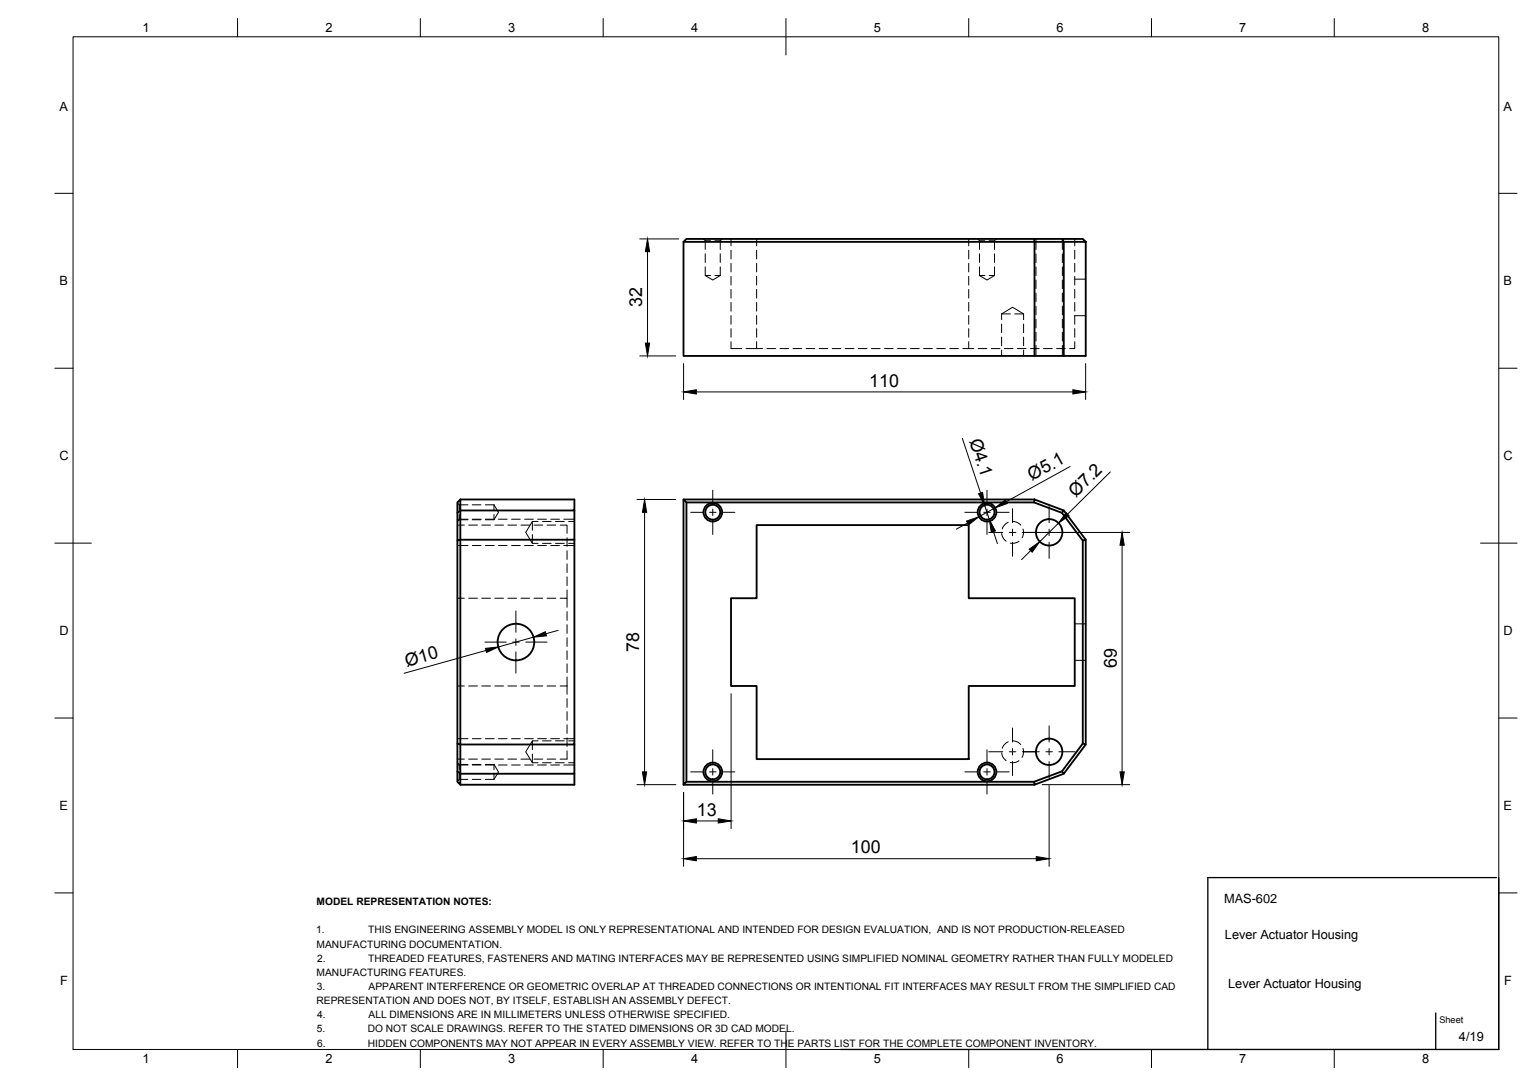
ISO-10303-21;
HEADER;
/* Generated by software containing ST-Developer
 * from STEP Tools, Inc. (www.steptools.com) 
 */

FILE_DESCRIPTION(
/* description */ (''),
/* implementation_level */ '2;1');

FILE_NAME(
/* name */ 'Lever Actuator Housing.step',
/* time_stamp */ '2026-10-15T14:42:47-07:00',
/* author */ (''),
/* organization */ (''),
/* preprocessor_version */ 'ST-DEVELOPER v20.2',
/* originating_system */ 'Autodesk Translation Framework v15.15.0.0',
/* authorisation */ '');

FILE_SCHEMA (('AUTOMOTIVE_DESIGN { 1 0 10303 214 3 1 1 }'));
ENDSEC;

DATA;
#10=MECHANICAL_DESIGN_GEOMETRIC_PRESENTATION_REPRESENTATION('',(#235),#85789);
#153=CONICAL_SURFACE('',#10323,0.1025,1.02974425867665);
#154=CONICAL_SURFACE('',#10327,0.255,0.785398163397446);
#155=CONICAL_SURFACE('',#10328,0.1025,1.02974425867665);
#156=CONICAL_SURFACE('',#10332,0.255,0.785398163397448);
#157=CONICAL_SURFACE('',#10333,0.1025,1.02974425867665);
#158=CONICAL_SURFACE('',#10337,0.255,0.785398163397446);
#159=CONICAL_SURFACE('',#10338,0.1025,1.02974425867665);
#160=CONICAL_SURFACE('',#10342,0.255,0.785398163397448);
#161=CONICAL_SURFACE('',#10343,0.15,1.02974425867665);
#162=CONICAL_SURFACE('',#10347,0.15,1.02974425867665);
#199=SHAPE_REPRESENTATION_RELATIONSHIP('SRR','None',#85864,#217);
#217=ADVANCED_BREP_SHAPE_REPRESENTATION('',(#253),#85772);
#235=STYLED_ITEM('',(#85963),#253);
#253=MANIFOLD_SOLID_BREP('Body1',#9882);
#398=FACE_BOUND('',#3084,.T.);
#399=FACE_BOUND('',#3085,.T.);
#400=FACE_BOUND('',#3086,.T.);
#401=FACE_BOUND('',#3087,.T.);
#402=FACE_BOUND('',#3088,.T.);
#403=FACE_BOUND('',#3089,.T.);
#404=FACE_BOUND('',#3090,.T.);
#405=FACE_BOUND('',#3114,.T.);
#406=FACE_BOUND('',#3126,.T.);
#407=FACE_BOUND('',#3130,.T.);
#408=FACE_BOUND('',#3131,.T.);
#409=FACE_BOUND('',#3132,.T.);
#410=FACE_BOUND('',#3133,.T.);
#1013=PLANE('',#10304);
#1014=PLANE('',#10305);
#1015=PLANE('',#10306);
#1016=PLANE('',#10307);
#1017=PLANE('',#10308);
#1018=PLANE('',#10309);
#1019=PLANE('',#10310);
#1020=PLANE('',#10311);
#1021=PLANE('',#10312);
#1022=PLANE('',#10313);
#1023=PLANE('',#10314);
#1024=PLANE('',#10315);
#1025=PLANE('',#10316);
#1026=PLANE('',#10358);
#1027=PLANE('',#10359);
#1028=PLANE('',#10360);
#1029=PLANE('',#10361);
#1030=PLANE('',#10362);
#1031=PLANE('',#10363);
#1032=PLANE('',#10364);
#1033=PLANE('',#10365);
#1034=PLANE('',#10366);
#1035=PLANE('',#10367);
#1036=PLANE('',#10368);
#1037=PLANE('',#10369);
#1038=PLANE('',#10370);
#1039=PLANE('',#10371);
#1040=PLANE('',#10372);
#1041=PLANE('',#10373);
#1042=PLANE('',#10374);
#1043=PLANE('',#10375);
#1262=LINE('',#23334,#1798);
#1263=LINE('',#23336,#1799);
#1264=LINE('',#23338,#1800);
#1265=LINE('',#23339,#1801);
#1266=LINE('',#23342,#1802);
#1267=LINE('',#23344,#1803);
#1268=LINE('',#23345,#1804);
#1269=LINE('',#23348,#1805);
#1270=LINE('',#23350,#1806);
#1271=LINE('',#23351,#1807);
#1272=LINE('',#23354,#1808);
#1273=LINE('',#23356,#1809);
#1274=LINE('',#23357,#1810);
#1275=LINE('',#23360,#1811);
#1276=LINE('',#23362,#1812);
#1277=LINE('',#23363,#1813);
#1278=LINE('',#23366,#1814);
#1279=LINE('',#23368,#1815);
#1280=LINE('',#23369,#1816);
#1281=LINE('',#23372,#1817);
#1282=LINE('',#23374,#1818);
#1283=LINE('',#23375,#1819);
#1284=LINE('',#23377,#1820);
#1285=LINE('',#23378,#1821);
#1286=LINE('',#23381,#1822);
#1287=LINE('',#23383,#1823);
#1288=LINE('',#23384,#1824);
#1289=LINE('',#23387,#1825);
#1290=LINE('',#23388,#1826);
#1291=LINE('',#23391,#1827);
#1292=LINE('',#23392,#1828);
#1293=LINE('',#23395,#1829);
#1294=LINE('',#23396,#1830);
#1295=LINE('',#23400,#1831);
#1296=LINE('',#23402,#1832);
#1297=LINE('',#23404,#1833);
#1298=LINE('',#23406,#1834);
#1299=LINE('',#23408,#1835);
#1300=LINE('',#23410,#1836);
#1301=LINE('',#23412,#1837);
#1302=LINE('',#23414,#1838);
#1303=LINE('',#23416,#1839);
#1304=LINE('',#23418,#1840);
#1305=LINE('',#23420,#1841);
#1306=LINE('',#23421,#1842);
#1307=LINE('',#23437,#1843);
#1308=LINE('',#23441,#1844);
#1309=LINE('',#23444,#1845);
#1310=LINE('',#23448,#1846);
#1311=LINE('',#23452,#1847);
#1312=LINE('',#23455,#1848);
#1313=LINE('',#23459,#1849);
#1314=LINE('',#23463,#1850);
#1315=LINE('',#23466,#1851);
#1316=LINE('',#23470,#1852);
#1317=LINE('',#23474,#1853);
#1318=LINE('',#23477,#1854);
#1319=LINE('',#23481,#1855);
#1320=LINE('',#23485,#1856);
#1321=LINE('',#23490,#1857);
#1322=LINE('',#23494,#1858);
#1323=LINE('',#23499,#1859);
#1324=LINE('',#23503,#1860);
#1325=LINE('',#23508,#1861);
#1326=LINE('',#23512,#1862);
#1327=LINE('',#23514,#1863);
#1328=LINE('',#23515,#1864);
#1329=LINE('',#23518,#1865);
#1330=LINE('',#23519,#1866);
#1331=LINE('',#23522,#1867);
#1332=LINE('',#23523,#1868);
#1333=LINE('',#23526,#1869);
#1334=LINE('',#23527,#1870);
#1335=LINE('',#23530,#1871);
#1336=LINE('',#23531,#1872);
#1337=LINE('',#23534,#1873);
#1338=LINE('',#23535,#1874);
#1339=LINE('',#23538,#1875);
#1340=LINE('',#23539,#1876);
#1341=LINE('',#23542,#1877);
#1342=LINE('',#23543,#1878);
#1343=LINE('',#23546,#1879);
#1344=LINE('',#23547,#1880);
#1345=LINE('',#23550,#1881);
#1346=LINE('',#23551,#1882);
#1347=LINE('',#23554,#1883);
#1348=LINE('',#23555,#1884);
#1349=LINE('',#23557,#1885);
#1350=LINE('',#23561,#1886);
#1351=LINE('',#23562,#1887);
#1352=LINE('',#23565,#1888);
#1353=LINE('',#23566,#1889);
#1354=LINE('',#23569,#1890);
#1355=LINE('',#23570,#1891);
#1356=LINE('',#23572,#1892);
#1798=VECTOR('',#11436,1.);
#1799=VECTOR('',#11437,1.);
#1800=VECTOR('',#11438,1.);
#1801=VECTOR('',#11439,0.999999999999999);
#1802=VECTOR('',#11442,1.);
#1803=VECTOR('',#11443,1.);
#1804=VECTOR('',#11444,1.);
#1805=VECTOR('',#11447,1.);
#1806=VECTOR('',#11448,1.);
#1807=VECTOR('',#11449,1.);
#1808=VECTOR('',#11452,1.);
#1809=VECTOR('',#11453,1.);
#1810=VECTOR('',#11454,1.);
#1811=VECTOR('',#11457,1.);
#1812=VECTOR('',#11458,1.);
#1813=VECTOR('',#11459,1.);
#1814=VECTOR('',#11462,1.);
#1815=VECTOR('',#11463,1.);
#1816=VECTOR('',#11464,1.);
#1817=VECTOR('',#11467,1.);
#1818=VECTOR('',#11468,1.);
#1819=VECTOR('',#11469,1.);
#1820=VECTOR('',#11472,1.);
#1821=VECTOR('',#11473,1.);
#1822=VECTOR('',#11476,1.);
#1823=VECTOR('',#11477,1.);
#1824=VECTOR('',#11478,1.);
#1825=VECTOR('',#11481,1.);
#1826=VECTOR('',#11482,1.);
#1827=VECTOR('',#11485,1.);
#1828=VECTOR('',#11486,1.);
#1829=VECTOR('',#11489,1.);
#1830=VECTOR('',#11490,1.);
#1831=VECTOR('',#11493,1.);
#1832=VECTOR('',#11494,1.);
#1833=VECTOR('',#11495,1.);
#1834=VECTOR('',#11496,1.);
#1835=VECTOR('',#11497,1.);
#1836=VECTOR('',#11498,1.);
#1837=VECTOR('',#11499,1.);
#1838=VECTOR('',#11500,1.);
#1839=VECTOR('',#11501,1.);
#1840=VECTOR('',#11502,1.);
#1841=VECTOR('',#11503,1.);
#1842=VECTOR('',#11504,1.);
#1843=VECTOR('',#11519,0.1025);
#1844=VECTOR('',#11524,0.205);
#1845=VECTOR('',#11529,0.255);
#1846=VECTOR('',#11532,0.1025);
#1847=VECTOR('',#11537,0.205);
#1848=VECTOR('',#11542,0.255);
#1849=VECTOR('',#11545,0.1025);
#1850=VECTOR('',#11550,0.205);
#1851=VECTOR('',#11555,0.255);
#1852=VECTOR('',#11558,0.1025);
#1853=VECTOR('',#11563,0.205);
#1854=VECTOR('',#11568,0.255);
#1855=VECTOR('',#11571,0.15);
#1856=VECTOR('',#11576,0.3);
#1857=VECTOR('',#11581,0.15);
#1858=VECTOR('',#11586,0.3);
#1859=VECTOR('',#11593,0.36);
#1860=VECTOR('',#11598,0.36);
#1861=VECTOR('',#11603,0.5);
#1862=VECTOR('',#11608,1.);
#1863=VECTOR('',#11609,1.);
#1864=VECTOR('',#11610,1.);
#1865=VECTOR('',#11613,1.);
#1866=VECTOR('',#11614,1.);
#1867=VECTOR('',#11617,1.);
#1868=VECTOR('',#11618,1.);
#1869=VECTOR('',#11621,1.);
#1870=VECTOR('',#11622,1.);
#1871=VECTOR('',#11625,1.);
#1872=VECTOR('',#11626,1.);
#1873=VECTOR('',#11629,1.);
#1874=VECTOR('',#11630,1.);
#1875=VECTOR('',#11633,1.);
#1876=VECTOR('',#11634,1.);
#1877=VECTOR('',#11637,1.);
#1878=VECTOR('',#11638,1.);
#1879=VECTOR('',#11641,1.);
#1880=VECTOR('',#11642,1.);
#1881=VECTOR('',#11645,1.);
#1882=VECTOR('',#11646,1.);
#1883=VECTOR('',#11649,1.);
#1884=VECTOR('',#11650,1.);
#1885=VECTOR('',#11653,1.);
#1886=VECTOR('',#11658,1.);
#1887=VECTOR('',#11659,1.);
#1888=VECTOR('',#11662,1.);
#1889=VECTOR('',#11663,1.);
#1890=VECTOR('',#11666,1.);
#1891=VECTOR('',#11667,1.);
#1892=VECTOR('',#11670,1.);
#2295=CYLINDRICAL_SURFACE('',#10325,0.205);
#2296=CYLINDRICAL_SURFACE('',#10330,0.205);
#2297=CYLINDRICAL_SURFACE('',#10335,0.205);
#2298=CYLINDRICAL_SURFACE('',#10340,0.205);
#2299=CYLINDRICAL_SURFACE('',#10345,0.3);
#2300=CYLINDRICAL_SURFACE('',#10349,0.3);
#2301=CYLINDRICAL_SURFACE('',#10351,0.36);
#2302=CYLINDRICAL_SURFACE('',#10353,0.36);
#2303=CYLINDRICAL_SURFACE('',#10355,0.5);
#2558=FACE_OUTER_BOUND('',#3071,.T.);
#2559=FACE_OUTER_BOUND('',#3072,.T.);
#2560=FACE_OUTER_BOUND('',#3073,.T.);
#2561=FACE_OUTER_BOUND('',#3074,.T.);
#2562=FACE_OUTER_BOUND('',#3075,.T.);
#2563=FACE_OUTER_BOUND('',#3076,.T.);
#2564=FACE_OUTER_BOUND('',#3077,.T.);
#2565=FACE_OUTER_BOUND('',#3078,.T.);
#2566=FACE_OUTER_BOUND('',#3079,.T.);
#2567=FACE_OUTER_BOUND('',#3080,.T.);
#2568=FACE_OUTER_BOUND('',#3081,.T.);
#2569=FACE_OUTER_BOUND('',#3082,.T.);
#2570=FACE_OUTER_BOUND('',#3083,.T.);
#2571=FACE_OUTER_BOUND('',#3091,.T.);
#2572=FACE_OUTER_BOUND('',#3092,.T.);
#2573=FACE_OUTER_BOUND('',#3093,.T.);
#2574=FACE_OUTER_BOUND('',#3094,.T.);
#2575=FACE_OUTER_BOUND('',#3095,.T.);
#2576=FACE_OUTER_BOUND('',#3096,.T.);
#2577=FACE_OUTER_BOUND('',#3097,.T.);
#2578=FACE_OUTER_BOUND('',#3098,.T.);
#2579=FACE_OUTER_BOUND('',#3099,.T.);
#2580=FACE_OUTER_BOUND('',#3100,.T.);
#2581=FACE_OUTER_BOUND('',#3101,.T.);
#2582=FACE_OUTER_BOUND('',#3102,.T.);
#2583=FACE_OUTER_BOUND('',#3103,.T.);
#2584=FACE_OUTER_BOUND('',#3104,.T.);
#2585=FACE_OUTER_BOUND('',#3105,.T.);
#2586=FACE_OUTER_BOUND('',#3106,.T.);
#2587=FACE_OUTER_BOUND('',#3107,.T.);
#2588=FACE_OUTER_BOUND('',#3108,.T.);
#2589=FACE_OUTER_BOUND('',#3109,.T.);
#2590=FACE_OUTER_BOUND('',#3110,.T.);
#2591=FACE_OUTER_BOUND('',#3111,.T.);
#2592=FACE_OUTER_BOUND('',#3112,.T.);
#2593=FACE_OUTER_BOUND('',#3113,.T.);
#2594=FACE_OUTER_BOUND('',#3115,.T.);
#2595=FACE_OUTER_BOUND('',#3116,.T.);
#2596=FACE_OUTER_BOUND('',#3117,.T.);
#2597=FACE_OUTER_BOUND('',#3118,.T.);
#2598=FACE_OUTER_BOUND('',#3119,.T.);
#2599=FACE_OUTER_BOUND('',#3120,.T.);
#2600=FACE_OUTER_BOUND('',#3121,.T.);
#2601=FACE_OUTER_BOUND('',#3122,.T.);
#2602=FACE_OUTER_BOUND('',#3123,.T.);
#2603=FACE_OUTER_BOUND('',#3124,.T.);
#2604=FACE_OUTER_BOUND('',#3125,.T.);
#2605=FACE_OUTER_BOUND('',#3127,.T.);
#2606=FACE_OUTER_BOUND('',#3128,.T.);
#2607=FACE_OUTER_BOUND('',#3129,.T.);
#3071=EDGE_LOOP('',(#7179,#7180,#7181,#7182));
#3072=EDGE_LOOP('',(#7183,#7184,#7185,#7186));
#3073=EDGE_LOOP('',(#7187,#7188,#7189,#7190));
#3074=EDGE_LOOP('',(#7191,#7192,#7193,#7194));
#3075=EDGE_LOOP('',(#7195,#7196,#7197,#7198));
#3076=EDGE_LOOP('',(#7199,#7200,#7201,#7202));
#3077=EDGE_LOOP('',(#7203,#7204,#7205,#7206));
#3078=EDGE_LOOP('',(#7207,#7208,#7209,#7210));
#3079=EDGE_LOOP('',(#7211,#7212,#7213,#7214));
#3080=EDGE_LOOP('',(#7215,#7216,#7217,#7218));
#3081=EDGE_LOOP('',(#7219,#7220,#7221,#7222));
#3082=EDGE_LOOP('',(#7223,#7224,#7225,#7226));
#3083=EDGE_LOOP('',(#7227,#7228,#7229,#7230,#7231,#7232,#7233,#7234));
#3084=EDGE_LOOP('',(#7235,#7236,#7237,#7238,#7239,#7240,#7241,#7242,#7243,
#7244,#7245,#7246));
#3085=EDGE_LOOP('',(#7247));
#3086=EDGE_LOOP('',(#7248));
#3087=EDGE_LOOP('',(#7249));
#3088=EDGE_LOOP('',(#7250));
#3089=EDGE_LOOP('',(#7251));
#3090=EDGE_LOOP('',(#7252));
#3091=EDGE_LOOP('',(#7253,#7254,#7255));
#3092=EDGE_LOOP('',(#7256,#7257,#7258,#7259));
#3093=EDGE_LOOP('',(#7260,#7261,#7262,#7263));
#3094=EDGE_LOOP('',(#7264,#7265,#7266));
#3095=EDGE_LOOP('',(#7267,#7268,#7269,#7270));
#3096=EDGE_LOOP('',(#7271,#7272,#7273,#7274));
#3097=EDGE_LOOP('',(#7275,#7276,#7277));
#3098=EDGE_LOOP('',(#7278,#7279,#7280,#7281));
#3099=EDGE_LOOP('',(#7282,#7283,#7284,#7285));
#3100=EDGE_LOOP('',(#7286,#7287,#7288));
#3101=EDGE_LOOP('',(#7289,#7290,#7291,#7292));
#3102=EDGE_LOOP('',(#7293,#7294,#7295,#7296));
#3103=EDGE_LOOP('',(#7297,#7298,#7299));
#3104=EDGE_LOOP('',(#7300,#7301,#7302,#7303));
#3105=EDGE_LOOP('',(#7304,#7305,#7306));
#3106=EDGE_LOOP('',(#7307,#7308,#7309,#7310));
#3107=EDGE_LOOP('',(#7311,#7312,#7313,#7314));
#3108=EDGE_LOOP('',(#7315,#7316,#7317,#7318));
#3109=EDGE_LOOP('',(#7319,#7320,#7321,#7322));
#3110=EDGE_LOOP('',(#7323,#7324,#7325,#7326));
#3111=EDGE_LOOP('',(#7327,#7328,#7329,#7330));
#3112=EDGE_LOOP('',(#7331,#7332,#7333,#7334));
#3113=EDGE_LOOP('',(#7335,#7336,#7337,#7338));
#3114=EDGE_LOOP('',(#7339));
#3115=EDGE_LOOP('',(#7340,#7341,#7342,#7343));
#3116=EDGE_LOOP('',(#7344,#7345,#7346,#7347));
#3117=EDGE_LOOP('',(#7348,#7349,#7350,#7351));
#3118=EDGE_LOOP('',(#7352,#7353,#7354,#7355));
#3119=EDGE_LOOP('',(#7356,#7357,#7358,#7359));
#3120=EDGE_LOOP('',(#7360,#7361,#7362,#7363));
#3121=EDGE_LOOP('',(#7364,#7365,#7366,#7367));
#3122=EDGE_LOOP('',(#7368,#7369,#7370,#7371));
#3123=EDGE_LOOP('',(#7372,#7373,#7374,#7375,#7376,#7377,#7378,#7379,#7380,
#7381,#7382,#7383));
#3124=EDGE_LOOP('',(#7384,#7385,#7386,#7387));
#3125=EDGE_LOOP('',(#7388,#7389,#7390,#7391));
#3126=EDGE_LOOP('',(#7392));
#3127=EDGE_LOOP('',(#7393,#7394,#7395,#7396));
#3128=EDGE_LOOP('',(#7397,#7398,#7399,#7400));
#3129=EDGE_LOOP('',(#7401,#7402,#7403,#7404,#7405,#7406,#7407,#7408));
#3130=EDGE_LOOP('',(#7409));
#3131=EDGE_LOOP('',(#7410));
#3132=EDGE_LOOP('',(#7411));
#3133=EDGE_LOOP('',(#7412));
#3626=CIRCLE('',#10317,0.36);
#3627=CIRCLE('',#10318,0.36);
#3628=CIRCLE('',#10319,0.255);
#3629=CIRCLE('',#10320,0.255);
#3630=CIRCLE('',#10321,0.255);
#3631=CIRCLE('',#10322,0.255);
#3632=CIRCLE('',#10324,0.205);
#3633=CIRCLE('',#10326,0.205);
#3634=CIRCLE('',#10329,0.205);
#3635=CIRCLE('',#10331,0.205);
#3636=CIRCLE('',#10334,0.205);
#3637=CIRCLE('',#10336,0.205);
#3638=CIRCLE('',#10339,0.205);
#3639=CIRCLE('',#10341,0.205);
#3640=CIRCLE('',#10344,0.3);
#3641=CIRCLE('',#10346,0.3);
#3642=CIRCLE('',#10348,0.3);
#3643=CIRCLE('',#10350,0.3);
#3644=CIRCLE('',#10352,0.36);
#3645=CIRCLE('',#10354,0.36);
#3646=CIRCLE('',#10356,0.5);
#3647=CIRCLE('',#10357,0.5);
#4123=VERTEX_POINT('',#23332);
#4124=VERTEX_POINT('',#23333);
#4125=VERTEX_POINT('',#23335);
#4126=VERTEX_POINT('',#23337);
#4127=VERTEX_POINT('',#23341);
#4128=VERTEX_POINT('',#23343);
#4129=VERTEX_POINT('',#23347);
#4130=VERTEX_POINT('',#23349);
#4131=VERTEX_POINT('',#23353);
#4132=VERTEX_POINT('',#23355);
#4133=VERTEX_POINT('',#23359);
#4134=VERTEX_POINT('',#23361);
#4135=VERTEX_POINT('',#23365);
#4136=VERTEX_POINT('',#23367);
#4137=VERTEX_POINT('',#23371);
#4138=VERTEX_POINT('',#23373);
#4139=VERTEX_POINT('',#23380);
#4140=VERTEX_POINT('',#23382);
#4141=VERTEX_POINT('',#23386);
#4142=VERTEX_POINT('',#23390);
#4143=VERTEX_POINT('',#23394);
#4144=VERTEX_POINT('',#23398);
#4145=VERTEX_POINT('',#23399);
#4146=VERTEX_POINT('',#23401);
#4147=VERTEX_POINT('',#23403);
#4148=VERTEX_POINT('',#23405);
#4149=VERTEX_POINT('',#23407);
#4150=VERTEX_POINT('',#23409);
#4151=VERTEX_POINT('',#23411);
#4152=VERTEX_POINT('',#23413);
#4153=VERTEX_POINT('',#23415);
#4154=VERTEX_POINT('',#23417);
#4155=VERTEX_POINT('',#23419);
#4156=VERTEX_POINT('',#23422);
#4157=VERTEX_POINT('',#23424);
#4158=VERTEX_POINT('',#23426);
#4159=VERTEX_POINT('',#23428);
#4160=VERTEX_POINT('',#23430);
#4161=VERTEX_POINT('',#23432);
#4162=VERTEX_POINT('',#23435);
#4163=VERTEX_POINT('',#23436);
#4164=VERTEX_POINT('',#23440);
#4165=VERTEX_POINT('',#23446);
#4166=VERTEX_POINT('',#23447);
#4167=VERTEX_POINT('',#23451);
#4168=VERTEX_POINT('',#23457);
#4169=VERTEX_POINT('',#23458);
#4170=VERTEX_POINT('',#23462);
#4171=VERTEX_POINT('',#23468);
#4172=VERTEX_POINT('',#23469);
#4173=VERTEX_POINT('',#23473);
#4174=VERTEX_POINT('',#23479);
#4175=VERTEX_POINT('',#23480);
#4176=VERTEX_POINT('',#23484);
#4177=VERTEX_POINT('',#23488);
#4178=VERTEX_POINT('',#23489);
#4179=VERTEX_POINT('',#23493);
#4180=VERTEX_POINT('',#23497);
#4181=VERTEX_POINT('',#23501);
#4182=VERTEX_POINT('',#23505);
#4183=VERTEX_POINT('',#23507);
#4184=VERTEX_POINT('',#23511);
#4185=VERTEX_POINT('',#23513);
#4186=VERTEX_POINT('',#23517);
#4187=VERTEX_POINT('',#23521);
#4188=VERTEX_POINT('',#23525);
#4189=VERTEX_POINT('',#23529);
#4190=VERTEX_POINT('',#23533);
#4191=VERTEX_POINT('',#23537);
#4192=VERTEX_POINT('',#23541);
#4193=VERTEX_POINT('',#23545);
#4194=VERTEX_POINT('',#23549);
#4195=VERTEX_POINT('',#23553);
#4196=VERTEX_POINT('',#23560);
#4197=VERTEX_POINT('',#23564);
#4198=VERTEX_POINT('',#23568);
#5317=EDGE_CURVE('',#4123,#4124,#1262,.T.);
#5318=EDGE_CURVE('',#4124,#4125,#1263,.T.);
#5319=EDGE_CURVE('',#4125,#4126,#1264,.T.);
#5320=EDGE_CURVE('',#4123,#4126,#1265,.T.);
#5321=EDGE_CURVE('',#4124,#4127,#1266,.T.);
#5322=EDGE_CURVE('',#4127,#4128,#1267,.T.);
#5323=EDGE_CURVE('',#4128,#4125,#1268,.T.);
#5324=EDGE_CURVE('',#4127,#4129,#1269,.T.);
#5325=EDGE_CURVE('',#4129,#4130,#1270,.T.);
#5326=EDGE_CURVE('',#4130,#4128,#1271,.T.);
#5327=EDGE_CURVE('',#4129,#4131,#1272,.T.);
#5328=EDGE_CURVE('',#4131,#4132,#1273,.T.);
#5329=EDGE_CURVE('',#4132,#4130,#1274,.T.);
#5330=EDGE_CURVE('',#4131,#4133,#1275,.T.);
#5331=EDGE_CURVE('',#4133,#4134,#1276,.T.);
#5332=EDGE_CURVE('',#4134,#4132,#1277,.T.);
#5333=EDGE_CURVE('',#4135,#4134,#1278,.T.);
#5334=EDGE_CURVE('',#4133,#4136,#1279,.T.);
#5335=EDGE_CURVE('',#4136,#4135,#1280,.T.);
#5336=EDGE_CURVE('',#4137,#4135,#1281,.T.);
#5337=EDGE_CURVE('',#4136,#4138,#1282,.T.);
#5338=EDGE_CURVE('',#4138,#4137,#1283,.T.);
#5339=EDGE_CURVE('',#4126,#4137,#1284,.T.);
#5340=EDGE_CURVE('',#4138,#4123,#1285,.T.);
#5341=EDGE_CURVE('',#4139,#4135,#1286,.T.);
#5342=EDGE_CURVE('',#4140,#4139,#1287,.T.);
#5343=EDGE_CURVE('',#4140,#4134,#1288,.T.);
#5344=EDGE_CURVE('',#4141,#4137,#1289,.T.);
#5345=EDGE_CURVE('',#4139,#4141,#1290,.T.);
#5346=EDGE_CURVE('',#4142,#4126,#1291,.T.);
#5347=EDGE_CURVE('',#4141,#4142,#1292,.T.);
#5348=EDGE_CURVE('',#4143,#4125,#1293,.T.);
#5349=EDGE_CURVE('',#4142,#4143,#1294,.T.);
#5350=EDGE_CURVE('',#4144,#4145,#1295,.T.);
#5351=EDGE_CURVE('',#4145,#4146,#1296,.T.);
#5352=EDGE_CURVE('',#4146,#4147,#1297,.T.);
#5353=EDGE_CURVE('',#4147,#4148,#1298,.T.);
#5354=EDGE_CURVE('',#4148,#4149,#1299,.T.);
#5355=EDGE_CURVE('',#4149,#4150,#1300,.T.);
#5356=EDGE_CURVE('',#4150,#4151,#1301,.T.);
#5357=EDGE_CURVE('',#4151,#4152,#1302,.T.);
#5358=EDGE_CURVE('',#4152,#4153,#1303,.T.);
#5359=EDGE_CURVE('',#4153,#4154,#1304,.T.);
#5360=EDGE_CURVE('',#4154,#4155,#1305,.T.);
#5361=EDGE_CURVE('',#4155,#4144,#1306,.T.);
#5362=EDGE_CURVE('',#4156,#4156,#3626,.T.);
#5363=EDGE_CURVE('',#4157,#4157,#3627,.T.);
#5364=EDGE_CURVE('',#4158,#4158,#3628,.T.);
#5365=EDGE_CURVE('',#4159,#4159,#3629,.T.);
#5366=EDGE_CURVE('',#4160,#4160,#3630,.T.);
#5367=EDGE_CURVE('',#4161,#4161,#3631,.T.);
#5368=EDGE_CURVE('',#4162,#4163,#1307,.T.);
#5369=EDGE_CURVE('',#4163,#4163,#3632,.T.);
#5370=EDGE_CURVE('',#4163,#4164,#1308,.T.);
#5371=EDGE_CURVE('',#4164,#4164,#3633,.T.);
#5372=EDGE_CURVE('',#4164,#4161,#1309,.T.);
#5373=EDGE_CURVE('',#4165,#4166,#1310,.T.);
#5374=EDGE_CURVE('',#4166,#4166,#3634,.T.);
#5375=EDGE_CURVE('',#4166,#4167,#1311,.T.);
#5376=EDGE_CURVE('',#4167,#4167,#3635,.T.);
#5377=EDGE_CURVE('',#4167,#4160,#1312,.T.);
#5378=EDGE_CURVE('',#4168,#4169,#1313,.T.);
#5379=EDGE_CURVE('',#4169,#4169,#3636,.T.);
#5380=EDGE_CURVE('',#4169,#4170,#1314,.T.);
#5381=EDGE_CURVE('',#4170,#4170,#3637,.T.);
#5382=EDGE_CURVE('',#4170,#4159,#1315,.T.);
#5383=EDGE_CURVE('',#4171,#4172,#1316,.T.);
#5384=EDGE_CURVE('',#4172,#4172,#3638,.T.);
#5385=EDGE_CURVE('',#4172,#4173,#1317,.T.);
#5386=EDGE_CURVE('',#4173,#4173,#3639,.T.);
#5387=EDGE_CURVE('',#4173,#4158,#1318,.T.);
#5388=EDGE_CURVE('',#4174,#4175,#1319,.T.);
#5389=EDGE_CURVE('',#4175,#4175,#3640,.T.);
#5390=EDGE_CURVE('',#4175,#4176,#1320,.T.);
#5391=EDGE_CURVE('',#4176,#4176,#3641,.T.);
#5392=EDGE_CURVE('',#4177,#4178,#1321,.T.);
#5393=EDGE_CURVE('',#4178,#4178,#3642,.T.);
#5394=EDGE_CURVE('',#4178,#4179,#1322,.T.);
#5395=EDGE_CURVE('',#4179,#4179,#3643,.T.);
#5396=EDGE_CURVE('',#4180,#4180,#3644,.T.);
#5397=EDGE_CURVE('',#4180,#4157,#1323,.T.);
#5398=EDGE_CURVE('',#4181,#4181,#3645,.T.);
#5399=EDGE_CURVE('',#4181,#4156,#1324,.T.);
#5400=EDGE_CURVE('',#4182,#4182,#3646,.T.);
#5401=EDGE_CURVE('',#4182,#4183,#1325,.T.);
#5402=EDGE_CURVE('',#4183,#4183,#3647,.T.);
#5403=EDGE_CURVE('',#4144,#4184,#1326,.T.);
#5404=EDGE_CURVE('',#4184,#4185,#1327,.T.);
#5405=EDGE_CURVE('',#4145,#4185,#1328,.T.);
#5406=EDGE_CURVE('',#4155,#4186,#1329,.T.);
#5407=EDGE_CURVE('',#4186,#4184,#1330,.T.);
#5408=EDGE_CURVE('',#4154,#4187,#1331,.T.);
#5409=EDGE_CURVE('',#4187,#4186,#1332,.T.);
#5410=EDGE_CURVE('',#4153,#4188,#1333,.T.);
#5411=EDGE_CURVE('',#4188,#4187,#1334,.T.);
#5412=EDGE_CURVE('',#4152,#4189,#1335,.T.);
#5413=EDGE_CURVE('',#4189,#4188,#1336,.T.);
#5414=EDGE_CURVE('',#4151,#4190,#1337,.T.);
#5415=EDGE_CURVE('',#4190,#4189,#1338,.T.);
#5416=EDGE_CURVE('',#4150,#4191,#1339,.T.);
#5417=EDGE_CURVE('',#4191,#4190,#1340,.T.);
#5418=EDGE_CURVE('',#4149,#4192,#1341,.T.);
#5419=EDGE_CURVE('',#4192,#4191,#1342,.T.);
#5420=EDGE_CURVE('',#4148,#4193,#1343,.T.);
#5421=EDGE_CURVE('',#4193,#4192,#1344,.T.);
#5422=EDGE_CURVE('',#4147,#4194,#1345,.T.);
#5423=EDGE_CURVE('',#4194,#4193,#1346,.T.);
#5424=EDGE_CURVE('',#4146,#4195,#1347,.T.);
#5425=EDGE_CURVE('',#4195,#4194,#1348,.T.);
#5426=EDGE_CURVE('',#4185,#4195,#1349,.T.);
#5427=EDGE_CURVE('',#4196,#4128,#1350,.T.);
#5428=EDGE_CURVE('',#4143,#4196,#1351,.T.);
#5429=EDGE_CURVE('',#4197,#4130,#1352,.T.);
#5430=EDGE_CURVE('',#4196,#4197,#1353,.T.);
#5431=EDGE_CURVE('',#4198,#4132,#1354,.T.);
#5432=EDGE_CURVE('',#4197,#4198,#1355,.T.);
#5433=EDGE_CURVE('',#4198,#4140,#1356,.T.);
#7179=ORIENTED_EDGE('',*,*,#5317,.T.);
#7180=ORIENTED_EDGE('',*,*,#5318,.T.);
#7181=ORIENTED_EDGE('',*,*,#5319,.T.);
#7182=ORIENTED_EDGE('',*,*,#5320,.F.);
#7183=ORIENTED_EDGE('',*,*,#5321,.T.);
#7184=ORIENTED_EDGE('',*,*,#5322,.T.);
#7185=ORIENTED_EDGE('',*,*,#5323,.T.);
#7186=ORIENTED_EDGE('',*,*,#5318,.F.);
#7187=ORIENTED_EDGE('',*,*,#5324,.T.);
#7188=ORIENTED_EDGE('',*,*,#5325,.T.);
#7189=ORIENTED_EDGE('',*,*,#5326,.T.);
#7190=ORIENTED_EDGE('',*,*,#5322,.F.);
#7191=ORIENTED_EDGE('',*,*,#5327,.T.);
#7192=ORIENTED_EDGE('',*,*,#5328,.T.);
#7193=ORIENTED_EDGE('',*,*,#5329,.T.);
#7194=ORIENTED_EDGE('',*,*,#5325,.F.);
#7195=ORIENTED_EDGE('',*,*,#5330,.T.);
#7196=ORIENTED_EDGE('',*,*,#5331,.T.);
#7197=ORIENTED_EDGE('',*,*,#5332,.T.);
#7198=ORIENTED_EDGE('',*,*,#5328,.F.);
#7199=ORIENTED_EDGE('',*,*,#5333,.T.);
#7200=ORIENTED_EDGE('',*,*,#5331,.F.);
#7201=ORIENTED_EDGE('',*,*,#5334,.T.);
#7202=ORIENTED_EDGE('',*,*,#5335,.T.);
#7203=ORIENTED_EDGE('',*,*,#5336,.T.);
#7204=ORIENTED_EDGE('',*,*,#5335,.F.);
#7205=ORIENTED_EDGE('',*,*,#5337,.T.);
#7206=ORIENTED_EDGE('',*,*,#5338,.T.);
#7207=ORIENTED_EDGE('',*,*,#5339,.T.);
#7208=ORIENTED_EDGE('',*,*,#5338,.F.);
#7209=ORIENTED_EDGE('',*,*,#5340,.T.);
#7210=ORIENTED_EDGE('',*,*,#5320,.T.);
#7211=ORIENTED_EDGE('',*,*,#5333,.F.);
#7212=ORIENTED_EDGE('',*,*,#5341,.F.);
#7213=ORIENTED_EDGE('',*,*,#5342,.F.);
#7214=ORIENTED_EDGE('',*,*,#5343,.T.);
#7215=ORIENTED_EDGE('',*,*,#5336,.F.);
#7216=ORIENTED_EDGE('',*,*,#5344,.F.);
#7217=ORIENTED_EDGE('',*,*,#5345,.F.);
#7218=ORIENTED_EDGE('',*,*,#5341,.T.);
#7219=ORIENTED_EDGE('',*,*,#5339,.F.);
#7220=ORIENTED_EDGE('',*,*,#5346,.F.);
#7221=ORIENTED_EDGE('',*,*,#5347,.F.);
#7222=ORIENTED_EDGE('',*,*,#5344,.T.);
#7223=ORIENTED_EDGE('',*,*,#5319,.F.);
#7224=ORIENTED_EDGE('',*,*,#5348,.F.);
#7225=ORIENTED_EDGE('',*,*,#5349,.F.);
#7226=ORIENTED_EDGE('',*,*,#5346,.T.);
#7227=ORIENTED_EDGE('',*,*,#5317,.F.);
#7228=ORIENTED_EDGE('',*,*,#5340,.F.);
#7229=ORIENTED_EDGE('',*,*,#5337,.F.);
#7230=ORIENTED_EDGE('',*,*,#5334,.F.);
#7231=ORIENTED_EDGE('',*,*,#5330,.F.);
#7232=ORIENTED_EDGE('',*,*,#5327,.F.);
#7233=ORIENTED_EDGE('',*,*,#5324,.F.);
#7234=ORIENTED_EDGE('',*,*,#5321,.F.);
#7235=ORIENTED_EDGE('',*,*,#5350,.T.);
#7236=ORIENTED_EDGE('',*,*,#5351,.T.);
#7237=ORIENTED_EDGE('',*,*,#5352,.T.);
#7238=ORIENTED_EDGE('',*,*,#5353,.T.);
#7239=ORIENTED_EDGE('',*,*,#5354,.T.);
#7240=ORIENTED_EDGE('',*,*,#5355,.T.);
#7241=ORIENTED_EDGE('',*,*,#5356,.T.);
#7242=ORIENTED_EDGE('',*,*,#5357,.T.);
#7243=ORIENTED_EDGE('',*,*,#5358,.T.);
#7244=ORIENTED_EDGE('',*,*,#5359,.T.);
#7245=ORIENTED_EDGE('',*,*,#5360,.T.);
#7246=ORIENTED_EDGE('',*,*,#5361,.T.);
#7247=ORIENTED_EDGE('',*,*,#5362,.T.);
#7248=ORIENTED_EDGE('',*,*,#5363,.T.);
#7249=ORIENTED_EDGE('',*,*,#5364,.T.);
#7250=ORIENTED_EDGE('',*,*,#5365,.T.);
#7251=ORIENTED_EDGE('',*,*,#5366,.T.);
#7252=ORIENTED_EDGE('',*,*,#5367,.T.);
#7253=ORIENTED_EDGE('',*,*,#5368,.T.);
#7254=ORIENTED_EDGE('',*,*,#5369,.T.);
#7255=ORIENTED_EDGE('',*,*,#5368,.F.);
#7256=ORIENTED_EDGE('',*,*,#5369,.F.);
#7257=ORIENTED_EDGE('',*,*,#5370,.T.);
#7258=ORIENTED_EDGE('',*,*,#5371,.T.);
#7259=ORIENTED_EDGE('',*,*,#5370,.F.);
#7260=ORIENTED_EDGE('',*,*,#5371,.F.);
#7261=ORIENTED_EDGE('',*,*,#5372,.T.);
#7262=ORIENTED_EDGE('',*,*,#5367,.F.);
#7263=ORIENTED_EDGE('',*,*,#5372,.F.);
#7264=ORIENTED_EDGE('',*,*,#5373,.T.);
#7265=ORIENTED_EDGE('',*,*,#5374,.T.);
#7266=ORIENTED_EDGE('',*,*,#5373,.F.);
#7267=ORIENTED_EDGE('',*,*,#5374,.F.);
#7268=ORIENTED_EDGE('',*,*,#5375,.T.);
#7269=ORIENTED_EDGE('',*,*,#5376,.T.);
#7270=ORIENTED_EDGE('',*,*,#5375,.F.);
#7271=ORIENTED_EDGE('',*,*,#5376,.F.);
#7272=ORIENTED_EDGE('',*,*,#5377,.T.);
#7273=ORIENTED_EDGE('',*,*,#5366,.F.);
#7274=ORIENTED_EDGE('',*,*,#5377,.F.);
#7275=ORIENTED_EDGE('',*,*,#5378,.T.);
#7276=ORIENTED_EDGE('',*,*,#5379,.T.);
#7277=ORIENTED_EDGE('',*,*,#5378,.F.);
#7278=ORIENTED_EDGE('',*,*,#5379,.F.);
#7279=ORIENTED_EDGE('',*,*,#5380,.T.);
#7280=ORIENTED_EDGE('',*,*,#5381,.T.);
#7281=ORIENTED_EDGE('',*,*,#5380,.F.);
#7282=ORIENTED_EDGE('',*,*,#5381,.F.);
#7283=ORIENTED_EDGE('',*,*,#5382,.T.);
#7284=ORIENTED_EDGE('',*,*,#5365,.F.);
#7285=ORIENTED_EDGE('',*,*,#5382,.F.);
#7286=ORIENTED_EDGE('',*,*,#5383,.T.);
#7287=ORIENTED_EDGE('',*,*,#5384,.T.);
#7288=ORIENTED_EDGE('',*,*,#5383,.F.);
#7289=ORIENTED_EDGE('',*,*,#5384,.F.);
#7290=ORIENTED_EDGE('',*,*,#5385,.T.);
#7291=ORIENTED_EDGE('',*,*,#5386,.T.);
#7292=ORIENTED_EDGE('',*,*,#5385,.F.);
#7293=ORIENTED_EDGE('',*,*,#5386,.F.);
#7294=ORIENTED_EDGE('',*,*,#5387,.T.);
#7295=ORIENTED_EDGE('',*,*,#5364,.F.);
#7296=ORIENTED_EDGE('',*,*,#5387,.F.);
#7297=ORIENTED_EDGE('',*,*,#5388,.T.);
#7298=ORIENTED_EDGE('',*,*,#5389,.T.);
#7299=ORIENTED_EDGE('',*,*,#5388,.F.);
#7300=ORIENTED_EDGE('',*,*,#5389,.F.);
#7301=ORIENTED_EDGE('',*,*,#5390,.T.);
#7302=ORIENTED_EDGE('',*,*,#5391,.F.);
#7303=ORIENTED_EDGE('',*,*,#5390,.F.);
#7304=ORIENTED_EDGE('',*,*,#5392,.T.);
#7305=ORIENTED_EDGE('',*,*,#5393,.T.);
#7306=ORIENTED_EDGE('',*,*,#5392,.F.);
#7307=ORIENTED_EDGE('',*,*,#5393,.F.);
#7308=ORIENTED_EDGE('',*,*,#5394,.T.);
#7309=ORIENTED_EDGE('',*,*,#5395,.F.);
#7310=ORIENTED_EDGE('',*,*,#5394,.F.);
#7311=ORIENTED_EDGE('',*,*,#5396,.F.);
#7312=ORIENTED_EDGE('',*,*,#5397,.T.);
#7313=ORIENTED_EDGE('',*,*,#5363,.F.);
#7314=ORIENTED_EDGE('',*,*,#5397,.F.);
#7315=ORIENTED_EDGE('',*,*,#5398,.F.);
#7316=ORIENTED_EDGE('',*,*,#5399,.T.);
#7317=ORIENTED_EDGE('',*,*,#5362,.F.);
#7318=ORIENTED_EDGE('',*,*,#5399,.F.);
#7319=ORIENTED_EDGE('',*,*,#5400,.F.);
#7320=ORIENTED_EDGE('',*,*,#5401,.T.);
#7321=ORIENTED_EDGE('',*,*,#5402,.F.);
#7322=ORIENTED_EDGE('',*,*,#5401,.F.);
#7323=ORIENTED_EDGE('',*,*,#5350,.F.);
#7324=ORIENTED_EDGE('',*,*,#5403,.T.);
#7325=ORIENTED_EDGE('',*,*,#5404,.T.);
#7326=ORIENTED_EDGE('',*,*,#5405,.F.);
#7327=ORIENTED_EDGE('',*,*,#5361,.F.);
#7328=ORIENTED_EDGE('',*,*,#5406,.T.);
#7329=ORIENTED_EDGE('',*,*,#5407,.T.);
#7330=ORIENTED_EDGE('',*,*,#5403,.F.);
#7331=ORIENTED_EDGE('',*,*,#5360,.F.);
#7332=ORIENTED_EDGE('',*,*,#5408,.T.);
#7333=ORIENTED_EDGE('',*,*,#5409,.T.);
#7334=ORIENTED_EDGE('',*,*,#5406,.F.);
#7335=ORIENTED_EDGE('',*,*,#5359,.F.);
#7336=ORIENTED_EDGE('',*,*,#5410,.T.);
#7337=ORIENTED_EDGE('',*,*,#5411,.T.);
#7338=ORIENTED_EDGE('',*,*,#5408,.F.);
#7339=ORIENTED_EDGE('',*,*,#5402,.T.);
#7340=ORIENTED_EDGE('',*,*,#5358,.F.);
#7341=ORIENTED_EDGE('',*,*,#5412,.T.);
#7342=ORIENTED_EDGE('',*,*,#5413,.T.);
#7343=ORIENTED_EDGE('',*,*,#5410,.F.);
#7344=ORIENTED_EDGE('',*,*,#5357,.F.);
#7345=ORIENTED_EDGE('',*,*,#5414,.T.);
#7346=ORIENTED_EDGE('',*,*,#5415,.T.);
#7347=ORIENTED_EDGE('',*,*,#5412,.F.);
#7348=ORIENTED_EDGE('',*,*,#5356,.F.);
#7349=ORIENTED_EDGE('',*,*,#5416,.T.);
#7350=ORIENTED_EDGE('',*,*,#5417,.T.);
#7351=ORIENTED_EDGE('',*,*,#5414,.F.);
#7352=ORIENTED_EDGE('',*,*,#5355,.F.);
#7353=ORIENTED_EDGE('',*,*,#5418,.T.);
#7354=ORIENTED_EDGE('',*,*,#5419,.T.);
#7355=ORIENTED_EDGE('',*,*,#5416,.F.);
#7356=ORIENTED_EDGE('',*,*,#5354,.F.);
#7357=ORIENTED_EDGE('',*,*,#5420,.T.);
#7358=ORIENTED_EDGE('',*,*,#5421,.T.);
#7359=ORIENTED_EDGE('',*,*,#5418,.F.);
#7360=ORIENTED_EDGE('',*,*,#5353,.F.);
#7361=ORIENTED_EDGE('',*,*,#5422,.T.);
#7362=ORIENTED_EDGE('',*,*,#5423,.T.);
#7363=ORIENTED_EDGE('',*,*,#5420,.F.);
#7364=ORIENTED_EDGE('',*,*,#5352,.F.);
#7365=ORIENTED_EDGE('',*,*,#5424,.T.);
#7366=ORIENTED_EDGE('',*,*,#5425,.T.);
#7367=ORIENTED_EDGE('',*,*,#5422,.F.);
#7368=ORIENTED_EDGE('',*,*,#5351,.F.);
#7369=ORIENTED_EDGE('',*,*,#5405,.T.);
#7370=ORIENTED_EDGE('',*,*,#5426,.T.);
#7371=ORIENTED_EDGE('',*,*,#5424,.F.);
#7372=ORIENTED_EDGE('',*,*,#5426,.F.);
#7373=ORIENTED_EDGE('',*,*,#5404,.F.);
#7374=ORIENTED_EDGE('',*,*,#5407,.F.);
#7375=ORIENTED_EDGE('',*,*,#5409,.F.);
#7376=ORIENTED_EDGE('',*,*,#5411,.F.);
#7377=ORIENTED_EDGE('',*,*,#5413,.F.);
#7378=ORIENTED_EDGE('',*,*,#5415,.F.);
#7379=ORIENTED_EDGE('',*,*,#5417,.F.);
#7380=ORIENTED_EDGE('',*,*,#5419,.F.);
#7381=ORIENTED_EDGE('',*,*,#5421,.F.);
#7382=ORIENTED_EDGE('',*,*,#5423,.F.);
#7383=ORIENTED_EDGE('',*,*,#5425,.F.);
#7384=ORIENTED_EDGE('',*,*,#5323,.F.);
#7385=ORIENTED_EDGE('',*,*,#5427,.F.);
#7386=ORIENTED_EDGE('',*,*,#5428,.F.);
#7387=ORIENTED_EDGE('',*,*,#5348,.T.);
#7388=ORIENTED_EDGE('',*,*,#5326,.F.);
#7389=ORIENTED_EDGE('',*,*,#5429,.F.);
#7390=ORIENTED_EDGE('',*,*,#5430,.F.);
#7391=ORIENTED_EDGE('',*,*,#5427,.T.);
#7392=ORIENTED_EDGE('',*,*,#5400,.T.);
#7393=ORIENTED_EDGE('',*,*,#5329,.F.);
#7394=ORIENTED_EDGE('',*,*,#5431,.F.);
#7395=ORIENTED_EDGE('',*,*,#5432,.F.);
#7396=ORIENTED_EDGE('',*,*,#5429,.T.);
#7397=ORIENTED_EDGE('',*,*,#5332,.F.);
#7398=ORIENTED_EDGE('',*,*,#5343,.F.);
#7399=ORIENTED_EDGE('',*,*,#5433,.F.);
#7400=ORIENTED_EDGE('',*,*,#5431,.T.);
#7401=ORIENTED_EDGE('',*,*,#5433,.T.);
#7402=ORIENTED_EDGE('',*,*,#5342,.T.);
#7403=ORIENTED_EDGE('',*,*,#5345,.T.);
#7404=ORIENTED_EDGE('',*,*,#5347,.T.);
#7405=ORIENTED_EDGE('',*,*,#5349,.T.);
#7406=ORIENTED_EDGE('',*,*,#5428,.T.);
#7407=ORIENTED_EDGE('',*,*,#5430,.T.);
#7408=ORIENTED_EDGE('',*,*,#5432,.T.);
#7409=ORIENTED_EDGE('',*,*,#5391,.T.);
#7410=ORIENTED_EDGE('',*,*,#5395,.T.);
#7411=ORIENTED_EDGE('',*,*,#5396,.T.);
#7412=ORIENTED_EDGE('',*,*,#5398,.T.);
#9536=ADVANCED_FACE('',(#2558),#1013,.T.);
#9537=ADVANCED_FACE('',(#2559),#1014,.T.);
#9538=ADVANCED_FACE('',(#2560),#1015,.T.);
#9539=ADVANCED_FACE('',(#2561),#1016,.T.);
#9540=ADVANCED_FACE('',(#2562),#1017,.T.);
#9541=ADVANCED_FACE('',(#2563),#1018,.T.);
#9542=ADVANCED_FACE('',(#2564),#1019,.T.);
#9543=ADVANCED_FACE('',(#2565),#1020,.T.);
#9544=ADVANCED_FACE('',(#2566),#1021,.T.);
#9545=ADVANCED_FACE('',(#2567),#1022,.T.);
#9546=ADVANCED_FACE('',(#2568),#1023,.T.);
#9547=ADVANCED_FACE('',(#2569),#1024,.T.);
#9548=ADVANCED_FACE('',(#2570,#398,#399,#400,#401,#402,#403,#404),#1025,
 .T.);
#9549=ADVANCED_FACE('',(#2571),#153,.F.);
#9550=ADVANCED_FACE('',(#2572),#2295,.F.);
#9551=ADVANCED_FACE('',(#2573),#154,.F.);
#9552=ADVANCED_FACE('',(#2574),#155,.F.);
#9553=ADVANCED_FACE('',(#2575),#2296,.F.);
#9554=ADVANCED_FACE('',(#2576),#156,.F.);
#9555=ADVANCED_FACE('',(#2577),#157,.F.);
#9556=ADVANCED_FACE('',(#2578),#2297,.F.);
#9557=ADVANCED_FACE('',(#2579),#158,.F.);
#9558=ADVANCED_FACE('',(#2580),#159,.F.);
#9559=ADVANCED_FACE('',(#2581),#2298,.F.);
#9560=ADVANCED_FACE('',(#2582),#160,.F.);
#9561=ADVANCED_FACE('',(#2583),#161,.F.);
#9562=ADVANCED_FACE('',(#2584),#2299,.F.);
#9563=ADVANCED_FACE('',(#2585),#162,.F.);
#9564=ADVANCED_FACE('',(#2586),#2300,.F.);
#9565=ADVANCED_FACE('',(#2587),#2301,.F.);
#9566=ADVANCED_FACE('',(#2588),#2302,.F.);
#9567=ADVANCED_FACE('',(#2589),#2303,.F.);
#9568=ADVANCED_FACE('',(#2590),#1026,.F.);
#9569=ADVANCED_FACE('',(#2591),#1027,.F.);
#9570=ADVANCED_FACE('',(#2592),#1028,.F.);
#9571=ADVANCED_FACE('',(#2593,#405),#1029,.F.);
#9572=ADVANCED_FACE('',(#2594),#1030,.F.);
#9573=ADVANCED_FACE('',(#2595),#1031,.F.);
#9574=ADVANCED_FACE('',(#2596),#1032,.F.);
#9575=ADVANCED_FACE('',(#2597),#1033,.F.);
#9576=ADVANCED_FACE('',(#2598),#1034,.F.);
#9577=ADVANCED_FACE('',(#2599),#1035,.F.);
#9578=ADVANCED_FACE('',(#2600),#1036,.F.);
#9579=ADVANCED_FACE('',(#2601),#1037,.F.);
#9580=ADVANCED_FACE('',(#2602),#1038,.F.);
#9581=ADVANCED_FACE('',(#2603),#1039,.T.);
#9582=ADVANCED_FACE('',(#2604,#406),#1040,.T.);
#9583=ADVANCED_FACE('',(#2605),#1041,.T.);
#9584=ADVANCED_FACE('',(#2606),#1042,.T.);
#9585=ADVANCED_FACE('',(#2607,#407,#408,#409,#410),#1043,.F.);
#9882=CLOSED_SHELL('',(#9536,#9537,#9538,#9539,#9540,#9541,#9542,#9543,
#9544,#9545,#9546,#9547,#9548,#9549,#9550,#9551,#9552,#9553,#9554,#9555,
#9556,#9557,#9558,#9559,#9560,#9561,#9562,#9563,#9564,#9565,#9566,#9567,
#9568,#9569,#9570,#9571,#9572,#9573,#9574,#9575,#9576,#9577,#9578,#9579,
#9580,#9581,#9582,#9583,#9584,#9585));
#10303=AXIS2_PLACEMENT_3D('',#23330,#11432,#11433);
#10304=AXIS2_PLACEMENT_3D('',#23331,#11434,#11435);
#10305=AXIS2_PLACEMENT_3D('',#23340,#11440,#11441);
#10306=AXIS2_PLACEMENT_3D('',#23346,#11445,#11446);
#10307=AXIS2_PLACEMENT_3D('',#23352,#11450,#11451);
#10308=AXIS2_PLACEMENT_3D('',#23358,#11455,#11456);
#10309=AXIS2_PLACEMENT_3D('',#23364,#11460,#11461);
#10310=AXIS2_PLACEMENT_3D('',#23370,#11465,#11466);
#10311=AXIS2_PLACEMENT_3D('',#23376,#11470,#11471);
#10312=AXIS2_PLACEMENT_3D('',#23379,#11474,#11475);
#10313=AXIS2_PLACEMENT_3D('',#23385,#11479,#11480);
#10314=AXIS2_PLACEMENT_3D('',#23389,#11483,#11484);
#10315=AXIS2_PLACEMENT_3D('',#23393,#11487,#11488);
#10316=AXIS2_PLACEMENT_3D('',#23397,#11491,#11492);
#10317=AXIS2_PLACEMENT_3D('',#23423,#11505,#11506);
#10318=AXIS2_PLACEMENT_3D('',#23425,#11507,#11508);
#10319=AXIS2_PLACEMENT_3D('',#23427,#11509,#11510);
#10320=AXIS2_PLACEMENT_3D('',#23429,#11511,#11512);
#10321=AXIS2_PLACEMENT_3D('',#23431,#11513,#11514);
#10322=AXIS2_PLACEMENT_3D('',#23433,#11515,#11516);
#10323=AXIS2_PLACEMENT_3D('',#23434,#11517,#11518);
#10324=AXIS2_PLACEMENT_3D('',#23438,#11520,#11521);
#10325=AXIS2_PLACEMENT_3D('',#23439,#11522,#11523);
#10326=AXIS2_PLACEMENT_3D('',#23442,#11525,#11526);
#10327=AXIS2_PLACEMENT_3D('',#23443,#11527,#11528);
#10328=AXIS2_PLACEMENT_3D('',#23445,#11530,#11531);
#10329=AXIS2_PLACEMENT_3D('',#23449,#11533,#11534);
#10330=AXIS2_PLACEMENT_3D('',#23450,#11535,#11536);
#10331=AXIS2_PLACEMENT_3D('',#23453,#11538,#11539);
#10332=AXIS2_PLACEMENT_3D('',#23454,#11540,#11541);
#10333=AXIS2_PLACEMENT_3D('',#23456,#11543,#11544);
#10334=AXIS2_PLACEMENT_3D('',#23460,#11546,#11547);
#10335=AXIS2_PLACEMENT_3D('',#23461,#11548,#11549);
#10336=AXIS2_PLACEMENT_3D('',#23464,#11551,#11552);
#10337=AXIS2_PLACEMENT_3D('',#23465,#11553,#11554);
#10338=AXIS2_PLACEMENT_3D('',#23467,#11556,#11557);
#10339=AXIS2_PLACEMENT_3D('',#23471,#11559,#11560);
#10340=AXIS2_PLACEMENT_3D('',#23472,#11561,#11562);
#10341=AXIS2_PLACEMENT_3D('',#23475,#11564,#11565);
#10342=AXIS2_PLACEMENT_3D('',#23476,#11566,#11567);
#10343=AXIS2_PLACEMENT_3D('',#23478,#11569,#11570);
#10344=AXIS2_PLACEMENT_3D('',#23482,#11572,#11573);
#10345=AXIS2_PLACEMENT_3D('',#23483,#11574,#11575);
#10346=AXIS2_PLACEMENT_3D('',#23486,#11577,#11578);
#10347=AXIS2_PLACEMENT_3D('',#23487,#11579,#11580);
#10348=AXIS2_PLACEMENT_3D('',#23491,#11582,#11583);
#10349=AXIS2_PLACEMENT_3D('',#23492,#11584,#11585);
#10350=AXIS2_PLACEMENT_3D('',#23495,#11587,#11588);
#10351=AXIS2_PLACEMENT_3D('',#23496,#11589,#11590);
#10352=AXIS2_PLACEMENT_3D('',#23498,#11591,#11592);
#10353=AXIS2_PLACEMENT_3D('',#23500,#11594,#11595);
#10354=AXIS2_PLACEMENT_3D('',#23502,#11596,#11597);
#10355=AXIS2_PLACEMENT_3D('',#23504,#11599,#11600);
#10356=AXIS2_PLACEMENT_3D('',#23506,#11601,#11602);
#10357=AXIS2_PLACEMENT_3D('',#23509,#11604,#11605);
#10358=AXIS2_PLACEMENT_3D('',#23510,#11606,#11607);
#10359=AXIS2_PLACEMENT_3D('',#23516,#11611,#11612);
#10360=AXIS2_PLACEMENT_3D('',#23520,#11615,#11616);
#10361=AXIS2_PLACEMENT_3D('',#23524,#11619,#11620);
#10362=AXIS2_PLACEMENT_3D('',#23528,#11623,#11624);
#10363=AXIS2_PLACEMENT_3D('',#23532,#11627,#11628);
#10364=AXIS2_PLACEMENT_3D('',#23536,#11631,#11632);
#10365=AXIS2_PLACEMENT_3D('',#23540,#11635,#11636);
#10366=AXIS2_PLACEMENT_3D('',#23544,#11639,#11640);
#10367=AXIS2_PLACEMENT_3D('',#23548,#11643,#11644);
#10368=AXIS2_PLACEMENT_3D('',#23552,#11647,#11648);
#10369=AXIS2_PLACEMENT_3D('',#23556,#11651,#11652);
#10370=AXIS2_PLACEMENT_3D('',#23558,#11654,#11655);
#10371=AXIS2_PLACEMENT_3D('',#23559,#11656,#11657);
#10372=AXIS2_PLACEMENT_3D('',#23563,#11660,#11661);
#10373=AXIS2_PLACEMENT_3D('',#23567,#11664,#11665);
#10374=AXIS2_PLACEMENT_3D('',#23571,#11668,#11669);
#10375=AXIS2_PLACEMENT_3D('',#23573,#11671,#11672);
#11432=DIRECTION('axis',(0.,0.,1.));
#11433=DIRECTION('refdir',(1.,0.,0.));
#11434=DIRECTION('center_axis',(0.662084710881893,0.707106781186549,0.24828176658071));
#11435=DIRECTION('ref_axis',(0.351123441588392,-1.5422241502084E-16,-0.936329177569044));
#11436=DIRECTION('',(-0.351123441588392,0.,0.936329177569044));
#11437=DIRECTION('',(0.577350269189626,-0.692482572856324,0.432590514178192));
#11438=DIRECTION('',(0.351123441588392,0.,-0.936329177569044));
#11439=DIRECTION('',(0.701364677853665,-0.701364677853665,0.127181670528612));
#11440=DIRECTION('center_axis',(0.424264068711928,0.707106781186549,0.565685424949237));
#11441=DIRECTION('ref_axis',(0.8,-1.29618843440069E-16,-0.6));
#11442=DIRECTION('',(-0.8,0.,0.6));
#11443=DIRECTION('',(0.22941573387057,-0.688247201611684,0.688247201611684));
#11444=DIRECTION('',(0.8,0.,-0.6));
#11445=DIRECTION('center_axis',(0.,0.707106781186548,0.707106781186548));
#11446=DIRECTION('ref_axis',(1.,0.,0.));
#11447=DIRECTION('',(-1.,0.,0.));
#11448=DIRECTION('',(-0.229415733870552,-0.688247201611687,0.688247201611687));
#11449=DIRECTION('',(1.,0.,0.));
#11450=DIRECTION('center_axis',(-0.424264068711929,0.707106781186546,0.565685424949239));
#11451=DIRECTION('ref_axis',(0.8,-1.26358053862033E-16,0.6));
#11452=DIRECTION('',(-0.8,0.,-0.6));
#11453=DIRECTION('',(-0.57735026918963,-0.692482572856329,0.43259051417818));
#11454=DIRECTION('',(0.8,0.,0.6));
#11455=DIRECTION('center_axis',(-0.662084710881897,0.707106781186545,0.248281766580712));
#11456=DIRECTION('ref_axis',(0.351123441588392,-1.9741179685392E-16,0.936329177569044));
#11457=DIRECTION('',(-0.351123441588392,0.,-0.936329177569044));
#11458=DIRECTION('',(-0.701364677853667,-0.701364677853667,0.127181670528596));
#11459=DIRECTION('',(0.351123441588392,0.,0.936329177569044));
#11460=DIRECTION('center_axis',(-0.707106781186548,0.707106781186548,0.));
#11461=DIRECTION('ref_axis',(0.,0.,1.));
#11462=DIRECTION('',(0.,0.,1.));
#11463=DIRECTION('',(0.,0.,-1.));
#11464=DIRECTION('',(-0.577350269189626,-0.577350269189623,-0.577350269189629));
#11465=DIRECTION('center_axis',(0.,0.707106781186549,-0.707106781186547));
#11466=DIRECTION('ref_axis',(-1.,0.,0.));
#11467=DIRECTION('',(-1.,0.,0.));
#11468=DIRECTION('',(1.,0.,0.));
#11469=DIRECTION('',(0.577350269189625,-0.577350269189625,-0.577350269189627));
#11470=DIRECTION('center_axis',(0.707106781186548,0.707106781186548,0.));
#11471=DIRECTION('ref_axis',(0.,0.,-1.));
#11472=DIRECTION('',(0.,0.,-1.));
#11473=DIRECTION('',(0.,0.,1.));
#11474=DIRECTION('center_axis',(-1.,0.,0.));
#11475=DIRECTION('ref_axis',(0.,0.,1.));
#11476=DIRECTION('',(0.,1.,0.));
#11477=DIRECTION('',(0.,0.,-1.));
#11478=DIRECTION('',(0.,1.,0.));
#11479=DIRECTION('center_axis',(0.,0.,-1.));
#11480=DIRECTION('ref_axis',(-1.,0.,0.));
#11481=DIRECTION('',(0.,1.,0.));
#11482=DIRECTION('',(1.,0.,0.));
#11483=DIRECTION('center_axis',(1.,0.,0.));
#11484=DIRECTION('ref_axis',(0.,0.,-1.));
#11485=DIRECTION('',(0.,1.,0.));
#11486=DIRECTION('',(0.,0.,1.));
#11487=DIRECTION('center_axis',(0.936329177569044,0.,0.351123441588392));
#11488=DIRECTION('ref_axis',(0.351123441588392,0.,-0.936329177569044));
#11489=DIRECTION('',(0.,1.,0.));
#11490=DIRECTION('',(-0.351123441588392,0.,0.936329177569044));
#11491=DIRECTION('center_axis',(0.,1.,0.));
#11492=DIRECTION('ref_axis',(0.,0.,1.));
#11493=DIRECTION('',(0.,0.,-1.));
#11494=DIRECTION('',(1.,0.,0.));
#11495=DIRECTION('',(0.,0.,-1.));
#11496=DIRECTION('',(1.,0.,0.));
#11497=DIRECTION('',(0.,0.,1.));
#11498=DIRECTION('',(1.,0.,0.));
#11499=DIRECTION('',(0.,0.,1.));
#11500=DIRECTION('',(-1.,0.,0.));
#11501=DIRECTION('',(0.,0.,1.));
#11502=DIRECTION('',(-1.,0.,0.));
#11503=DIRECTION('',(0.,0.,-1.));
#11504=DIRECTION('',(-1.,0.,0.));
#11505=DIRECTION('center_axis',(0.,-1.,0.));
#11506=DIRECTION('ref_axis',(1.,0.,0.));
#11507=DIRECTION('center_axis',(0.,-1.,0.));
#11508=DIRECTION('ref_axis',(1.,0.,0.));
#11509=DIRECTION('center_axis',(0.,-1.,0.));
#11510=DIRECTION('ref_axis',(-1.,0.,0.));
#11511=DIRECTION('center_axis',(0.,-1.,0.));
#11512=DIRECTION('ref_axis',(-1.,0.,0.));
#11513=DIRECTION('center_axis',(0.,-1.,0.));
#11514=DIRECTION('ref_axis',(-1.,0.,0.));
#11515=DIRECTION('center_axis',(0.,-1.,0.));
#11516=DIRECTION('ref_axis',(-1.,0.,0.));
#11517=DIRECTION('center_axis',(0.,1.,0.));
#11518=DIRECTION('ref_axis',(-1.,0.,0.));
#11519=DIRECTION('',(0.85716730070211,0.515038074910058,-1.04972719113862E-16));
#11520=DIRECTION('center_axis',(0.,1.,0.));
#11521=DIRECTION('ref_axis',(1.,0.,0.));
#11522=DIRECTION('center_axis',(0.,1.,0.));
#11523=DIRECTION('ref_axis',(-1.,0.,0.));
#11524=DIRECTION('',(0.,1.,0.));
#11525=DIRECTION('center_axis',(0.,1.,0.));
#11526=DIRECTION('ref_axis',(1.,0.,0.));
#11527=DIRECTION('center_axis',(0.,1.,0.));
#11528=DIRECTION('ref_axis',(-1.,0.,0.));
#11529=DIRECTION('',(0.707106781186546,0.707106781186549,-8.65956056235491E-17));
#11530=DIRECTION('center_axis',(0.,1.,0.));
#11531=DIRECTION('ref_axis',(-1.,0.,0.));
#11532=DIRECTION('',(0.85716730070211,0.515038074910058,-1.04972719113862E-16));
#11533=DIRECTION('center_axis',(0.,1.,0.));
#11534=DIRECTION('ref_axis',(1.,0.,0.));
#11535=DIRECTION('center_axis',(0.,1.,0.));
#11536=DIRECTION('ref_axis',(-1.,0.,0.));
#11537=DIRECTION('',(0.,1.,0.));
#11538=DIRECTION('center_axis',(0.,1.,0.));
#11539=DIRECTION('ref_axis',(1.,0.,0.));
#11540=DIRECTION('center_axis',(0.,1.,0.));
#11541=DIRECTION('ref_axis',(-1.,0.,0.));
#11542=DIRECTION('',(0.707106781186547,0.707106781186548,-8.65956056235493E-17));
#11543=DIRECTION('center_axis',(0.,1.,0.));
#11544=DIRECTION('ref_axis',(-1.,0.,0.));
#11545=DIRECTION('',(0.85716730070211,0.515038074910058,-1.04972719113862E-16));
#11546=DIRECTION('center_axis',(0.,1.,0.));
#11547=DIRECTION('ref_axis',(1.,0.,0.));
#11548=DIRECTION('center_axis',(0.,1.,0.));
#11549=DIRECTION('ref_axis',(-1.,0.,0.));
#11550=DIRECTION('',(0.,1.,0.));
#11551=DIRECTION('center_axis',(0.,1.,0.));
#11552=DIRECTION('ref_axis',(1.,0.,0.));
#11553=DIRECTION('center_axis',(0.,1.,0.));
#11554=DIRECTION('ref_axis',(-1.,0.,0.));
#11555=DIRECTION('',(0.707106781186546,0.707106781186549,-8.65956056235491E-17));
#11556=DIRECTION('center_axis',(0.,1.,0.));
#11557=DIRECTION('ref_axis',(-1.,0.,0.));
#11558=DIRECTION('',(0.85716730070211,0.515038074910058,-1.04972719113862E-16));
#11559=DIRECTION('center_axis',(0.,1.,0.));
#11560=DIRECTION('ref_axis',(1.,0.,0.));
#11561=DIRECTION('center_axis',(0.,1.,0.));
#11562=DIRECTION('ref_axis',(-1.,0.,0.));
#11563=DIRECTION('',(0.,1.,0.));
#11564=DIRECTION('center_axis',(0.,1.,0.));
#11565=DIRECTION('ref_axis',(1.,0.,0.));
#11566=DIRECTION('center_axis',(0.,1.,0.));
#11567=DIRECTION('ref_axis',(-1.,0.,0.));
#11568=DIRECTION('',(0.707106781186547,0.707106781186548,-8.65956056235493E-17));
#11569=DIRECTION('center_axis',(0.,-1.,0.));
#11570=DIRECTION('ref_axis',(1.,0.,0.));
#11571=DIRECTION('',(-0.85716730070211,-0.515038074910058,-1.04972719113862E-16));
#11572=DIRECTION('center_axis',(0.,-1.,0.));
#11573=DIRECTION('ref_axis',(1.,0.,0.));
#11574=DIRECTION('center_axis',(0.,-1.,0.));
#11575=DIRECTION('ref_axis',(1.,0.,0.));
#11576=DIRECTION('',(0.,-1.,0.));
#11577=DIRECTION('center_axis',(0.,1.,0.));
#11578=DIRECTION('ref_axis',(1.,0.,0.));
#11579=DIRECTION('center_axis',(0.,-1.,0.));
#11580=DIRECTION('ref_axis',(1.,0.,0.));
#11581=DIRECTION('',(-0.85716730070211,-0.515038074910058,-1.04972719113862E-16));
#11582=DIRECTION('center_axis',(0.,-1.,0.));
#11583=DIRECTION('ref_axis',(1.,0.,0.));
#11584=DIRECTION('center_axis',(0.,-1.,0.));
#11585=DIRECTION('ref_axis',(1.,0.,0.));
#11586=DIRECTION('',(0.,-1.,0.));
#11587=DIRECTION('center_axis',(0.,1.,0.));
#11588=DIRECTION('ref_axis',(1.,0.,0.));
#11589=DIRECTION('center_axis',(0.,1.,0.));
#11590=DIRECTION('ref_axis',(1.,0.,0.));
#11591=DIRECTION('center_axis',(0.,1.,0.));
#11592=DIRECTION('ref_axis',(1.,0.,0.));
#11593=DIRECTION('',(0.,1.,0.));
#11594=DIRECTION('center_axis',(0.,1.,0.));
#11595=DIRECTION('ref_axis',(1.,0.,0.));
#11596=DIRECTION('center_axis',(0.,1.,0.));
#11597=DIRECTION('ref_axis',(1.,0.,0.));
#11598=DIRECTION('',(0.,1.,0.));
#11599=DIRECTION('center_axis',(0.,0.,-1.));
#11600=DIRECTION('ref_axis',(1.,0.,0.));
#11601=DIRECTION('center_axis',(0.,0.,-1.));
#11602=DIRECTION('ref_axis',(1.,0.,0.));
#11603=DIRECTION('',(0.,0.,-1.));
#11604=DIRECTION('center_axis',(0.,0.,1.));
#11605=DIRECTION('ref_axis',(1.,0.,0.));
#11606=DIRECTION('center_axis',(-1.,0.,0.));
#11607=DIRECTION('ref_axis',(0.,0.,-1.));
#11608=DIRECTION('',(0.,-1.,0.));
#11609=DIRECTION('',(0.,0.,-1.));
#11610=DIRECTION('',(0.,-1.,0.));
#11611=DIRECTION('center_axis',(0.,0.,1.));
#11612=DIRECTION('ref_axis',(-1.,0.,0.));
#11613=DIRECTION('',(0.,-1.,0.));
#11614=DIRECTION('',(-1.,0.,0.));
#11615=DIRECTION('center_axis',(-1.,0.,0.));
#11616=DIRECTION('ref_axis',(0.,0.,-1.));
#11617=DIRECTION('',(0.,-1.,0.));
#11618=DIRECTION('',(0.,0.,-1.));
#11619=DIRECTION('center_axis',(0.,0.,1.));
#11620=DIRECTION('ref_axis',(-1.,0.,0.));
#11621=DIRECTION('',(0.,-1.,0.));
#11622=DIRECTION('',(-1.,0.,0.));
#11623=DIRECTION('center_axis',(1.,0.,0.));
#11624=DIRECTION('ref_axis',(0.,0.,1.));
#11625=DIRECTION('',(0.,-1.,0.));
#11626=DIRECTION('',(0.,0.,1.));
#11627=DIRECTION('center_axis',(0.,0.,1.));
#11628=DIRECTION('ref_axis',(-1.,0.,0.));
#11629=DIRECTION('',(0.,-1.,0.));
#11630=DIRECTION('',(-1.,0.,0.));
#11631=DIRECTION('center_axis',(1.,0.,0.));
#11632=DIRECTION('ref_axis',(0.,0.,1.));
#11633=DIRECTION('',(0.,-1.,0.));
#11634=DIRECTION('',(0.,0.,1.));
#11635=DIRECTION('center_axis',(0.,0.,-1.));
#11636=DIRECTION('ref_axis',(1.,0.,0.));
#11637=DIRECTION('',(0.,-1.,0.));
#11638=DIRECTION('',(1.,0.,0.));
#11639=DIRECTION('center_axis',(1.,0.,0.));
#11640=DIRECTION('ref_axis',(0.,0.,1.));
#11641=DIRECTION('',(0.,-1.,0.));
#11642=DIRECTION('',(0.,0.,1.));
#11643=DIRECTION('center_axis',(0.,0.,-1.));
#11644=DIRECTION('ref_axis',(1.,0.,0.));
#11645=DIRECTION('',(0.,-1.,0.));
#11646=DIRECTION('',(1.,0.,0.));
#11647=DIRECTION('center_axis',(-1.,0.,0.));
#11648=DIRECTION('ref_axis',(0.,0.,-1.));
#11649=DIRECTION('',(0.,-1.,0.));
#11650=DIRECTION('',(0.,0.,-1.));
#11651=DIRECTION('center_axis',(0.,0.,-1.));
#11652=DIRECTION('ref_axis',(1.,0.,0.));
#11653=DIRECTION('',(1.,0.,0.));
#11654=DIRECTION('center_axis',(0.,-1.,0.));
#11655=DIRECTION('ref_axis',(0.,0.,-1.));
#11656=DIRECTION('center_axis',(0.6,0.,0.8));
#11657=DIRECTION('ref_axis',(0.8,0.,-0.6));
#11658=DIRECTION('',(0.,1.,0.));
#11659=DIRECTION('',(-0.8,0.,0.6));
#11660=DIRECTION('center_axis',(0.,0.,1.));
#11661=DIRECTION('ref_axis',(1.,0.,0.));
#11662=DIRECTION('',(0.,1.,0.));
#11663=DIRECTION('',(-1.,0.,0.));
#11664=DIRECTION('center_axis',(-0.6,0.,0.8));
#11665=DIRECTION('ref_axis',(0.8,0.,0.6));
#11666=DIRECTION('',(0.,1.,0.));
#11667=DIRECTION('',(-0.8,0.,-0.6));
#11668=DIRECTION('center_axis',(-0.936329177569044,0.,0.351123441588392));
#11669=DIRECTION('ref_axis',(0.351123441588392,0.,0.936329177569044));
#11670=DIRECTION('',(-0.351123441588392,0.,-0.936329177569044));
#11671=DIRECTION('center_axis',(0.,1.,0.));
#11672=DIRECTION('ref_axis',(1.,0.,0.));
#23330=CARTESIAN_POINT('',(0.,0.,0.));
#23331=CARTESIAN_POINT('Origin',(4.14610847673285,3.66,10.5297906787748));
#23332=CARTESIAN_POINT('',(3.82,3.7,11.2854932334582));
#23333=CARTESIAN_POINT('',(3.53330081745645,3.7,12.0500243869077));
#23334=CARTESIAN_POINT('',(4.10865530963009,3.7,10.5157457411113));
#23335=CARTESIAN_POINT('',(3.6,3.62,12.1));
#23336=CARTESIAN_POINT('',(3.53330081745645,3.7,12.0500243869077));
#23337=CARTESIAN_POINT('',(3.9,3.62,11.3));
#23338=CARTESIAN_POINT('',(4.18356164383562,3.62,10.5438356164384));
#23339=CARTESIAN_POINT('',(3.82,3.7,11.2854932334582));
#23340=CARTESIAN_POINT('Origin',(3.2,3.66,12.35));
#23341=CARTESIAN_POINT('',(2.77333333333333,3.7,12.62));
#23342=CARTESIAN_POINT('',(3.176,3.7,12.318));
#23343=CARTESIAN_POINT('',(2.8,3.62,12.7));
#23344=CARTESIAN_POINT('',(2.77333333333333,3.7,12.62));
#23345=CARTESIAN_POINT('',(3.224,3.62,12.382));
#23346=CARTESIAN_POINT('Origin',(-1.4,3.66,12.66));
#23347=CARTESIAN_POINT('',(-2.77333333333333,3.7,12.62));
#23348=CARTESIAN_POINT('',(-1.4,3.7,12.62));
#23349=CARTESIAN_POINT('',(-2.8,3.62,12.7));
#23350=CARTESIAN_POINT('',(-2.77333333333333,3.7,12.62));
#23351=CARTESIAN_POINT('',(-1.4,3.62,12.7));
#23352=CARTESIAN_POINT('Origin',(-3.6,3.66,12.05));
#23353=CARTESIAN_POINT('',(-3.53330081745645,3.7,12.0500243869077));
#23354=CARTESIAN_POINT('',(-3.576,3.7,12.018));
#23355=CARTESIAN_POINT('',(-3.6,3.62,12.1));
#23356=CARTESIAN_POINT('',(-3.53330081745645,3.7,12.0500243869077));
#23357=CARTESIAN_POINT('',(-3.624,3.62,12.082));
#23358=CARTESIAN_POINT('Origin',(-4.29610847673285,3.66,10.1297906787748));
#23359=CARTESIAN_POINT('',(-3.82,3.7,11.2854932334582));
#23360=CARTESIAN_POINT('',(-4.25865530963009,3.7,10.1157457411113));
#23361=CARTESIAN_POINT('',(-3.9,3.62,11.3));
#23362=CARTESIAN_POINT('',(-3.82,3.7,11.2854932334582));
#23363=CARTESIAN_POINT('',(-4.33356164383562,3.62,10.1438356164384));
#23364=CARTESIAN_POINT('Origin',(-3.86,3.66,4.45));
#23365=CARTESIAN_POINT('',(-3.9,3.62,1.7));
#23366=CARTESIAN_POINT('',(-3.9,3.62,4.45));
#23367=CARTESIAN_POINT('',(-3.82,3.7,1.78));
#23368=CARTESIAN_POINT('',(-3.82,3.7,4.45));
#23369=CARTESIAN_POINT('',(-3.82,3.7,1.78));
#23370=CARTESIAN_POINT('Origin',(1.95,3.66,1.74));
#23371=CARTESIAN_POINT('',(3.9,3.62,1.7));
#23372=CARTESIAN_POINT('',(1.95,3.62,1.7));
#23373=CARTESIAN_POINT('',(3.82,3.7,1.78));
#23374=CARTESIAN_POINT('',(1.95,3.7,1.78));
#23375=CARTESIAN_POINT('',(3.82,3.7,1.78));
#23376=CARTESIAN_POINT('Origin',(3.86,3.66,9.25));
#23377=CARTESIAN_POINT('',(3.9,3.62,9.25));
#23378=CARTESIAN_POINT('',(3.82,3.7,9.25));
#23379=CARTESIAN_POINT('Origin',(-3.9,0.5,1.7));
#23380=CARTESIAN_POINT('',(-3.9,0.5,1.7));
#23381=CARTESIAN_POINT('',(-3.9,0.5,1.7));
#23382=CARTESIAN_POINT('',(-3.9,0.5,11.3));
#23383=CARTESIAN_POINT('',(-3.9,0.5,11.3));
#23384=CARTESIAN_POINT('',(-3.9,0.5,11.3));
#23385=CARTESIAN_POINT('Origin',(3.9,0.5,1.7));
#23386=CARTESIAN_POINT('',(3.9,0.5,1.7));
#23387=CARTESIAN_POINT('',(3.9,0.5,1.7));
#23388=CARTESIAN_POINT('',(-3.9,0.5,1.7));
#23389=CARTESIAN_POINT('Origin',(3.9,0.5,11.3));
#23390=CARTESIAN_POINT('',(3.9,0.5,11.3));
#23391=CARTESIAN_POINT('',(3.9,0.5,11.3));
#23392=CARTESIAN_POINT('',(3.9,0.5,1.7));
#23393=CARTESIAN_POINT('Origin',(3.6,0.5,12.1));
#23394=CARTESIAN_POINT('',(3.6,0.5,12.1));
#23395=CARTESIAN_POINT('',(3.6,0.5,12.1));
#23396=CARTESIAN_POINT('',(3.9,0.5,11.3));
#23397=CARTESIAN_POINT('Origin',(0.,3.7,7.2));
#23398=CARTESIAN_POINT('',(-3.2,3.7,9.5));
#23399=CARTESIAN_POINT('',(-3.2,3.7,3.7));
#23400=CARTESIAN_POINT('',(-3.2,3.7,8.35));
#23401=CARTESIAN_POINT('',(-1.2,3.7,3.7));
#23402=CARTESIAN_POINT('',(-1.6,3.7,3.7));
#23403=CARTESIAN_POINT('',(-1.2,3.7,3.));
#23404=CARTESIAN_POINT('',(-1.2,3.7,5.45));
#23405=CARTESIAN_POINT('',(1.2,3.7,3.));
#23406=CARTESIAN_POINT('',(-0.6,3.7,3.));
#23407=CARTESIAN_POINT('',(1.2,3.7,3.7));
#23408=CARTESIAN_POINT('',(1.2,3.7,5.1));
#23409=CARTESIAN_POINT('',(3.2,3.7,3.7));
#23410=CARTESIAN_POINT('',(0.6,3.7,3.7));
#23411=CARTESIAN_POINT('',(3.2,3.7,9.5));
#23412=CARTESIAN_POINT('',(3.2,3.7,5.45));
#23413=CARTESIAN_POINT('',(1.2,3.7,9.5));
#23414=CARTESIAN_POINT('',(1.6,3.7,9.5));
#23415=CARTESIAN_POINT('',(1.2,3.7,12.4));
#23416=CARTESIAN_POINT('',(1.2,3.7,8.35));
#23417=CARTESIAN_POINT('',(-1.2,3.7,12.4));
#23418=CARTESIAN_POINT('',(0.6,3.7,12.4));
#23419=CARTESIAN_POINT('',(-1.2,3.7,9.5));
#23420=CARTESIAN_POINT('',(-1.2,3.7,9.8));
#23421=CARTESIAN_POINT('',(-0.6,3.7,9.5));
#23422=CARTESIAN_POINT('',(-3.36,3.7,11.7));
#23423=CARTESIAN_POINT('Origin',(-3.,3.7,11.7));
#23424=CARTESIAN_POINT('',(2.64,3.7,11.7));
#23425=CARTESIAN_POINT('Origin',(3.,3.7,11.7));
#23426=CARTESIAN_POINT('',(3.805,3.7,2.5));
#23427=CARTESIAN_POINT('Origin',(3.55,3.7,2.5));
#23428=CARTESIAN_POINT('',(-3.295,3.7,2.5));
#23429=CARTESIAN_POINT('Origin',(-3.55,3.7,2.5));
#23430=CARTESIAN_POINT('',(3.805,3.7,10.));
#23431=CARTESIAN_POINT('Origin',(3.55,3.7,10.));
#23432=CARTESIAN_POINT('',(-3.295,3.7,10.));
#23433=CARTESIAN_POINT('Origin',(-3.55,3.7,10.));
#23434=CARTESIAN_POINT('Origin',(-3.55,2.63841178654968,10.));
#23435=CARTESIAN_POINT('',(-3.55,2.57682357309935,10.));
#23436=CARTESIAN_POINT('',(-3.345,2.7,10.));
#23437=CARTESIAN_POINT('',(-3.4475,2.63841178654968,10.));
#23438=CARTESIAN_POINT('Origin',(-3.55,2.7,10.));
#23439=CARTESIAN_POINT('Origin',(-3.55,3.175,10.));
#23440=CARTESIAN_POINT('',(-3.345,3.65,10.));
#23441=CARTESIAN_POINT('',(-3.345,3.175,10.));
#23442=CARTESIAN_POINT('Origin',(-3.55,3.65,10.));
#23443=CARTESIAN_POINT('Origin',(-3.55,3.7,10.));
#23444=CARTESIAN_POINT('',(-3.295,3.7,10.));
#23445=CARTESIAN_POINT('Origin',(3.55,2.63841178654968,10.));
#23446=CARTESIAN_POINT('',(3.55,2.57682357309935,10.));
#23447=CARTESIAN_POINT('',(3.755,2.7,10.));
#23448=CARTESIAN_POINT('',(3.6525,2.63841178654968,10.));
#23449=CARTESIAN_POINT('Origin',(3.55,2.7,10.));
#23450=CARTESIAN_POINT('Origin',(3.55,3.175,10.));
#23451=CARTESIAN_POINT('',(3.755,3.65,10.));
#23452=CARTESIAN_POINT('',(3.755,3.175,10.));
#23453=CARTESIAN_POINT('Origin',(3.55,3.65,10.));
#23454=CARTESIAN_POINT('Origin',(3.55,3.7,10.));
#23455=CARTESIAN_POINT('',(3.805,3.7,10.));
#23456=CARTESIAN_POINT('Origin',(-3.55,2.63841178654968,2.5));
#23457=CARTESIAN_POINT('',(-3.55,2.57682357309935,2.5));
#23458=CARTESIAN_POINT('',(-3.345,2.7,2.5));
#23459=CARTESIAN_POINT('',(-3.4475,2.63841178654968,2.5));
#23460=CARTESIAN_POINT('Origin',(-3.55,2.7,2.5));
#23461=CARTESIAN_POINT('Origin',(-3.55,3.175,2.5));
#23462=CARTESIAN_POINT('',(-3.345,3.65,2.5));
#23463=CARTESIAN_POINT('',(-3.345,3.175,2.5));
#23464=CARTESIAN_POINT('Origin',(-3.55,3.65,2.5));
#23465=CARTESIAN_POINT('Origin',(-3.55,3.7,2.5));
#23466=CARTESIAN_POINT('',(-3.295,3.7,2.5));
#23467=CARTESIAN_POINT('Origin',(3.55,2.63841178654968,2.5));
#23468=CARTESIAN_POINT('',(3.55,2.57682357309935,2.5));
#23469=CARTESIAN_POINT('',(3.755,2.7,2.5));
#23470=CARTESIAN_POINT('',(3.6525,2.63841178654968,2.5));
#23471=CARTESIAN_POINT('Origin',(3.55,2.7,2.5));
#23472=CARTESIAN_POINT('Origin',(3.55,3.175,2.5));
#23473=CARTESIAN_POINT('',(3.755,3.65,2.5));
#23474=CARTESIAN_POINT('',(3.755,3.175,2.5));
#23475=CARTESIAN_POINT('Origin',(3.55,3.65,2.5));
#23476=CARTESIAN_POINT('Origin',(3.55,3.7,2.5));
#23477=CARTESIAN_POINT('',(3.805,3.7,2.5));
#23478=CARTESIAN_POINT('Origin',(-3.,1.74012909285413,10.7));
#23479=CARTESIAN_POINT('',(-3.,1.83025818570827,10.7));
#23480=CARTESIAN_POINT('',(-3.3,1.65,10.7));
#23481=CARTESIAN_POINT('',(-3.15,1.74012909285413,10.7));
#23482=CARTESIAN_POINT('Origin',(-3.,1.65,10.7));
#23483=CARTESIAN_POINT('Origin',(-3.,1.05,10.7));
#23484=CARTESIAN_POINT('',(-3.3,0.5,10.7));
#23485=CARTESIAN_POINT('',(-3.3,1.05,10.7));
#23486=CARTESIAN_POINT('Origin',(-3.,0.5,10.7));
#23487=CARTESIAN_POINT('Origin',(3.,1.74012909285413,10.7));
#23488=CARTESIAN_POINT('',(3.,1.83025818570827,10.7));
#23489=CARTESIAN_POINT('',(2.7,1.65,10.7));
#23490=CARTESIAN_POINT('',(2.85,1.74012909285413,10.7));
#23491=CARTESIAN_POINT('Origin',(3.,1.65,10.7));
#23492=CARTESIAN_POINT('Origin',(3.,1.05,10.7));
#23493=CARTESIAN_POINT('',(2.7,0.5,10.7));
#23494=CARTESIAN_POINT('',(2.7,1.05,10.7));
#23495=CARTESIAN_POINT('Origin',(3.,0.5,10.7));
#23496=CARTESIAN_POINT('Origin',(3.,0.5,11.7));
#23497=CARTESIAN_POINT('',(2.64,0.5,11.7));
#23498=CARTESIAN_POINT('Origin',(3.,0.5,11.7));
#23499=CARTESIAN_POINT('',(2.64,0.5,11.7));
#23500=CARTESIAN_POINT('Origin',(-3.,0.5,11.7));
#23501=CARTESIAN_POINT('',(-3.36,0.5,11.7));
#23502=CARTESIAN_POINT('Origin',(-3.,0.5,11.7));
#23503=CARTESIAN_POINT('',(-3.36,0.5,11.7));
#23504=CARTESIAN_POINT('Origin',(0.,2.1,12.7));
#23505=CARTESIAN_POINT('',(-0.5,2.1,12.7));
#23506=CARTESIAN_POINT('Origin',(0.,2.1,12.7));
#23507=CARTESIAN_POINT('',(-0.5,2.1,12.4));
#23508=CARTESIAN_POINT('',(-0.5,2.1,12.7));
#23509=CARTESIAN_POINT('Origin',(0.,2.1,12.4));
#23510=CARTESIAN_POINT('Origin',(-3.2,3.7,9.5));
#23511=CARTESIAN_POINT('',(-3.2,0.7,9.5));
#23512=CARTESIAN_POINT('',(-3.2,3.7,9.5));
#23513=CARTESIAN_POINT('',(-3.2,0.7,3.7));
#23514=CARTESIAN_POINT('',(-3.2,0.7,9.5));
#23515=CARTESIAN_POINT('',(-3.2,3.7,3.7));
#23516=CARTESIAN_POINT('Origin',(-1.2,3.7,9.5));
#23517=CARTESIAN_POINT('',(-1.2,0.7,9.5));
#23518=CARTESIAN_POINT('',(-1.2,3.7,9.5));
#23519=CARTESIAN_POINT('',(-1.2,0.7,9.5));
#23520=CARTESIAN_POINT('Origin',(-1.2,3.7,12.4));
#23521=CARTESIAN_POINT('',(-1.2,0.7,12.4));
#23522=CARTESIAN_POINT('',(-1.2,3.7,12.4));
#23523=CARTESIAN_POINT('',(-1.2,0.7,12.4));
#23524=CARTESIAN_POINT('Origin',(1.2,3.7,12.4));
#23525=CARTESIAN_POINT('',(1.2,0.7,12.4));
#23526=CARTESIAN_POINT('',(1.2,3.7,12.4));
#23527=CARTESIAN_POINT('',(1.2,0.7,12.4));
#23528=CARTESIAN_POINT('Origin',(1.2,3.7,9.5));
#23529=CARTESIAN_POINT('',(1.2,0.7,9.5));
#23530=CARTESIAN_POINT('',(1.2,3.7,9.5));
#23531=CARTESIAN_POINT('',(1.2,0.7,9.5));
#23532=CARTESIAN_POINT('Origin',(3.2,3.7,9.5));
#23533=CARTESIAN_POINT('',(3.2,0.7,9.5));
#23534=CARTESIAN_POINT('',(3.2,3.7,9.5));
#23535=CARTESIAN_POINT('',(3.2,0.7,9.5));
#23536=CARTESIAN_POINT('Origin',(3.2,3.7,3.7));
#23537=CARTESIAN_POINT('',(3.2,0.7,3.7));
#23538=CARTESIAN_POINT('',(3.2,3.7,3.7));
#23539=CARTESIAN_POINT('',(3.2,0.7,3.7));
#23540=CARTESIAN_POINT('Origin',(1.2,3.7,3.7));
#23541=CARTESIAN_POINT('',(1.2,0.7,3.7));
#23542=CARTESIAN_POINT('',(1.2,3.7,3.7));
#23543=CARTESIAN_POINT('',(1.2,0.7,3.7));
#23544=CARTESIAN_POINT('Origin',(1.2,3.7,3.));
#23545=CARTESIAN_POINT('',(1.2,0.7,3.));
#23546=CARTESIAN_POINT('',(1.2,3.7,3.));
#23547=CARTESIAN_POINT('',(1.2,0.7,3.));
#23548=CARTESIAN_POINT('Origin',(-1.2,3.7,3.));
#23549=CARTESIAN_POINT('',(-1.2,0.7,3.));
#23550=CARTESIAN_POINT('',(-1.2,3.7,3.));
#23551=CARTESIAN_POINT('',(-1.2,0.7,3.));
#23552=CARTESIAN_POINT('Origin',(-1.2,3.7,3.7));
#23553=CARTESIAN_POINT('',(-1.2,0.7,3.7));
#23554=CARTESIAN_POINT('',(-1.2,3.7,3.7));
#23555=CARTESIAN_POINT('',(-1.2,0.7,3.7));
#23556=CARTESIAN_POINT('Origin',(-3.2,3.7,3.7));
#23557=CARTESIAN_POINT('',(-3.2,0.7,3.7));
#23558=CARTESIAN_POINT('Origin',(0.,0.7,7.7));
#23559=CARTESIAN_POINT('Origin',(2.8,0.5,12.7));
#23560=CARTESIAN_POINT('',(2.8,0.5,12.7));
#23561=CARTESIAN_POINT('',(2.8,0.5,12.7));
#23562=CARTESIAN_POINT('',(3.6,0.5,12.1));
#23563=CARTESIAN_POINT('Origin',(-2.8,0.5,12.7));
#23564=CARTESIAN_POINT('',(-2.8,0.5,12.7));
#23565=CARTESIAN_POINT('',(-2.8,0.5,12.7));
#23566=CARTESIAN_POINT('',(2.8,0.5,12.7));
#23567=CARTESIAN_POINT('Origin',(-3.6,0.5,12.1));
#23568=CARTESIAN_POINT('',(-3.6,0.5,12.1));
#23569=CARTESIAN_POINT('',(-3.6,0.5,12.1));
#23570=CARTESIAN_POINT('',(-2.8,0.5,12.7));
#23571=CARTESIAN_POINT('Origin',(-3.9,0.5,11.3));
#23572=CARTESIAN_POINT('',(-3.6,0.5,12.1));
#23573=CARTESIAN_POINT('Origin',(0.,0.5,7.2));
#85752=UNCERTAINTY_MEASURE_WITH_UNIT(LENGTH_MEASURE(0.001),#85790,
'DISTANCE_ACCURACY_VALUE',
'Maximum model space distance between geometric entities at asserted c
onnectivities');
#85769=UNCERTAINTY_MEASURE_WITH_UNIT(LENGTH_MEASURE(0.001),#85790,
'DISTANCE_ACCURACY_VALUE',
'Maximum model space distance between geometric entities at asserted c
onnectivities');
#85772=(
GEOMETRIC_REPRESENTATION_CONTEXT(3)
GLOBAL_UNCERTAINTY_ASSIGNED_CONTEXT((#85752))
GLOBAL_UNIT_ASSIGNED_CONTEXT((#85790,#85792,#85793))
REPRESENTATION_CONTEXT('','3D')
);
#85789=(
GEOMETRIC_REPRESENTATION_CONTEXT(3)
GLOBAL_UNCERTAINTY_ASSIGNED_CONTEXT((#85769))
GLOBAL_UNIT_ASSIGNED_CONTEXT((#85790,#85792,#85793))
REPRESENTATION_CONTEXT('','3D')
);
#85790=(
LENGTH_UNIT()
NAMED_UNIT(*)
SI_UNIT(.CENTI.,.METRE.)
);
#85792=(
NAMED_UNIT(*)
PLANE_ANGLE_UNIT()
SI_UNIT($,.RADIAN.)
);
#85793=(
NAMED_UNIT(*)
SI_UNIT($,.STERADIAN.)
SOLID_ANGLE_UNIT()
);
#85796=SHAPE_DEFINITION_REPRESENTATION(#85815,#85864);
#85815=PRODUCT_DEFINITION_SHAPE('',$,#85884);
#85864=SHAPE_REPRESENTATION('',(#10303),#85772);
#85881=PRODUCT_DEFINITION_CONTEXT('part definition',#85940,'design');
#85884=PRODUCT_DEFINITION('Lever Actuator Housing',
'Lever Actuator Housing',#85903,#85881);
#85903=PRODUCT_DEFINITION_FORMATION('',$,#85944);
#85940=APPLICATION_CONTEXT(
'Core Data for Automotive Mechanical Design Process');
#85941=PRODUCT_CONTEXT('part definition',#85940,'mechanical');
#85944=PRODUCT('Lever Actuator Housing','Lever Actuator Housing',$,(#85941));
#85963=PRESENTATION_STYLE_ASSIGNMENT((#85981));
#85981=SURFACE_STYLE_USAGE(.BOTH.,#85999);
#85999=SURFACE_SIDE_STYLE('',(#86017));
#86017=SURFACE_STYLE_FILL_AREA(#86035);
#86035=FILL_AREA_STYLE('Opaque(176,180,186)',(#86053));
#86053=FILL_AREA_STYLE_COLOUR('Opaque(176,180,186)',#86071);
#86071=COLOUR_RGB('Opaque(176,180,186)', 0.31764706, 0.68627451, 0.89019608);
ENDSEC;
END-ISO-10303-21;
